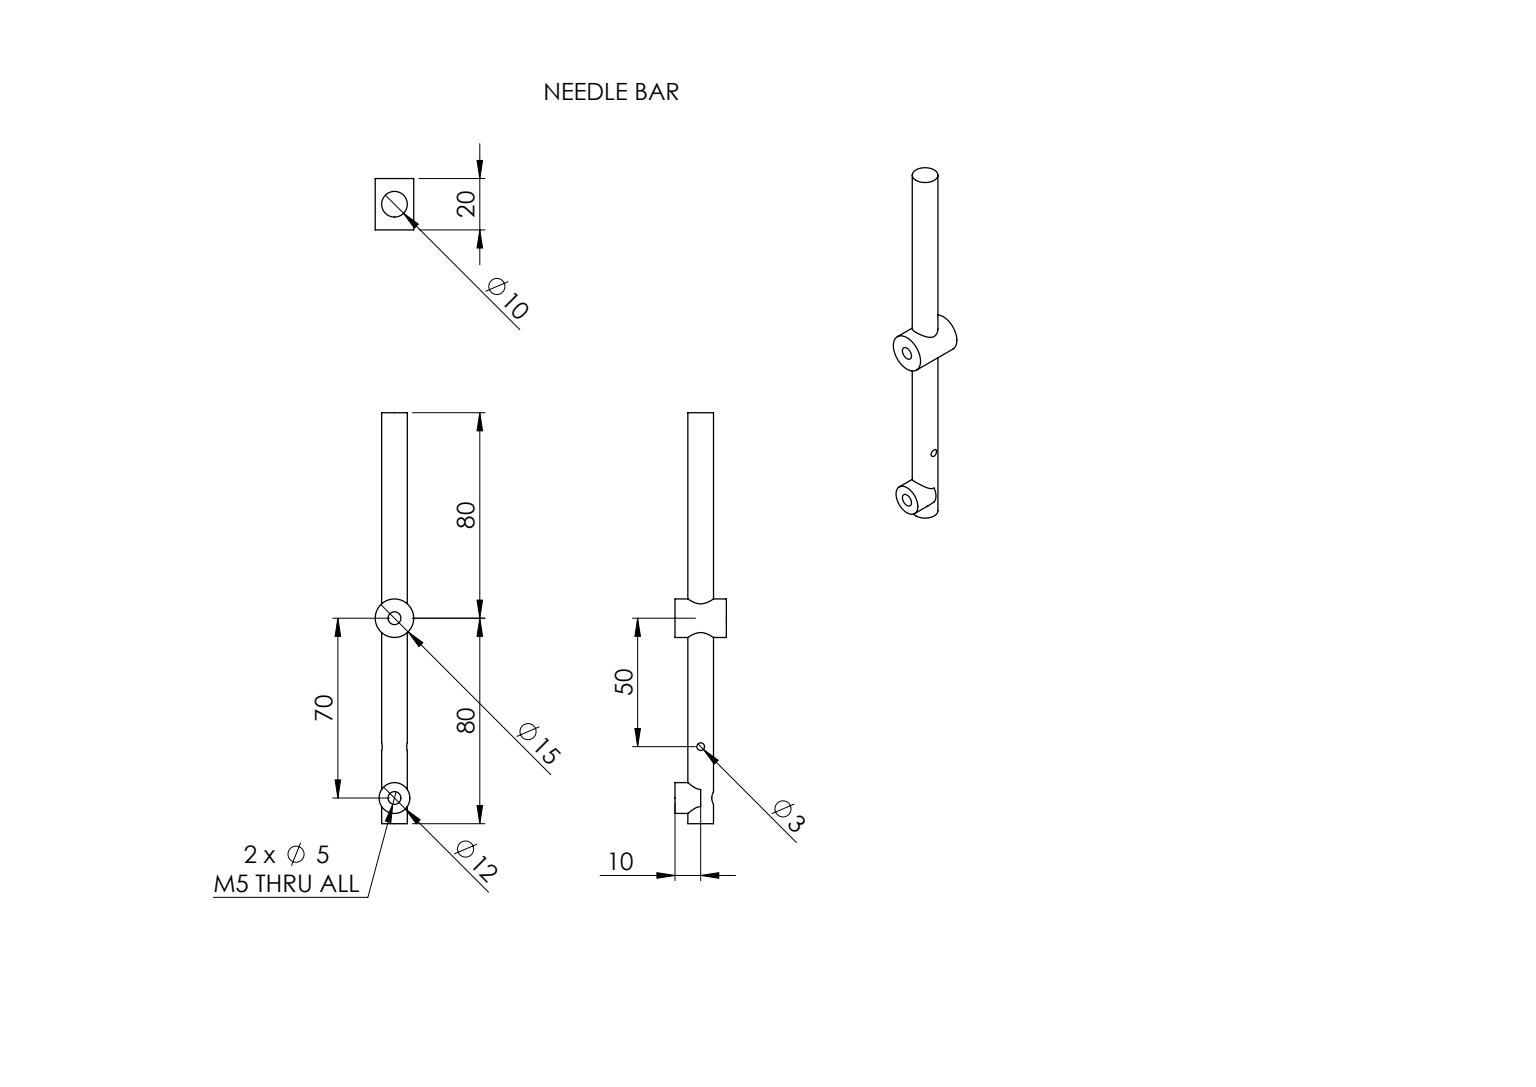
ISO-10303-21;
HEADER;
FILE_DESCRIPTION (('STEP AP214'),
    '1' );
FILE_NAME ('Needle Bar.step',
    '2026-10-25T11:00:22',
    ( '' ),
    ( '' ),
    'SwSTEP 2.0',
    'SolidWorks 2026',
    '' );
FILE_SCHEMA (( 'AUTOMOTIVE_DESIGN' ));
ENDSEC;

DATA;
#4=CARTESIAN_POINT ( 'NONE',  ( 4.999998311775604165, -51.49999437258534130, 0.09894250604207632804 ) ) ;
#5=SHAPE_DEFINITION_REPRESENTATION ( #2134, #457 ) ;
#6=CYLINDRICAL_SURFACE ( 'NONE', #1532, 4.999999999999999112 ) ;
#7=CARTESIAN_POINT ( 'NONE',  ( -0.1736799743064503798, -76.00000000000005684, 5.000000000000000000 ) ) ;
#8=UNCERTAINTY_MEASURE_WITH_UNIT (LENGTH_MEASURE( 1.000000000000000082E-05 ), #1107, 'distance_accuracy_value', 'NONE');
#17=CARTESIAN_POINT ( 'NONE',  ( 0.3311419820765648669, -72.48349571540411773, -4.991687326893459620 ) ) ;
#18=CARTESIAN_POINT ( 'NONE',  ( 2.499999999999999556, 3.061616997868382648E-16, 10.00000000000000000 ) ) ;
#21=CARTESIAN_POINT ( 'NONE',  ( 4.769696007084727185, -50.19647014491117432, 1.499999999999993339 ) ) ;
#22=ADVANCED_FACE ( 'NONE', ( #937 ), #2745, .F. ) ;
#24=CARTESIAN_POINT ( 'NONE',  ( -4.828212536628694984, -50.75366254478191053, 1.300578314244078992 ) ) ;
#26=CARTESIAN_POINT ( 'NONE',  ( 3.061616997868384127E-16, -72.50000000000001421, 2.500000000000000444 ) ) ;
#29=EDGE_LOOP ( 'NONE', ( #3142, #458 ) ) ;
#33=ORIENTED_EDGE ( 'NONE', *, *, #1677, .F. ) ;
#34=CARTESIAN_POINT ( 'NONE',  ( 4.871330634494102974, -50.99215130299450038, -1.129198576418441791 ) ) ;
#39=CARTESIAN_POINT ( 'NONE',  ( -3.982914377913044479, -74.49364316089672400, 3.038300766938668573 ) ) ;
#41=CARTESIAN_POINT ( 'NONE',  ( -7.500000000000000000, -50.00000000000000000, -1.500000000000006439 ) ) ;
#43=DIRECTION ( 'NONE',  ( 1.000000000000000000, -0.000000000000000000, -0.000000000000000000 ) ) ;
#46=DIRECTION ( 'NONE',  ( 0.000000000000000000, 1.000000000000000000, 0.000000000000000000 ) ) ;
#47=AXIS2_PLACEMENT_3D ( 'NONE', #892, #615, #1900 ) ;
#49=CARTESIAN_POINT ( 'NONE',  ( -6.610444160707455418E-15, -72.50000000000009948, -5.000000000000047962 ) ) ;
#51=CARTESIAN_POINT ( 'NONE',  ( 4.977204064302565456, -51.42262508310333402, -0.4855051584829146449 ) ) ;
#53=CIRCLE ( 'NONE', #2065, 4.999999999999999112 ) ;
#54=ADVANCED_FACE ( 'NONE', ( #463, #744 ), #700, .T. ) ;
#55=CARTESIAN_POINT ( 'NONE',  ( -0.3471650268615569246, -75.99247303379605967, 4.990975288187767589 ) ) ;
#57=CARTESIAN_POINT ( 'NONE',  ( 0.000000000000000000, 0.000000000000000000, 10.00000000000000000 ) ) ;
#59=EDGE_CURVE ( 'NONE', #1569, #129, #2568, .T. ) ;
#62=ORIENTED_EDGE ( 'NONE', *, *, #59, .F. ) ;
#63=CARTESIAN_POINT ( 'NONE',  ( 8.572527594031472993E-15, -70.00000000000000000, 10.00000000000000000 ) ) ;
#64=CARTESIAN_POINT ( 'NONE',  ( -2.499999999999995559, -70.00000000000000000, 0.000000000000000000 ) ) ;
#65=CARTESIAN_POINT ( 'NONE',  ( 4.964478897467096807, -5.622442520179988357, 0.6821754209311353678 ) ) ;
#68=CARTESIAN_POINT ( 'NONE',  ( -0.6778607859896496057, 7.476644527972223564, 4.965157125901431101 ) ) ;
#70=ORIENTED_EDGE ( 'NONE', *, *, #2414, .T. ) ;
#72=ADVANCED_FACE ( 'NONE', ( #1264 ), #1017, .F. ) ;
#79=CARTESIAN_POINT ( 'NONE',  ( 8.572527594031472993E-15, -70.00000000000000000, 10.00000000000000000 ) ) ;
#81=CARTESIAN_POINT ( 'NONE',  ( 4.966432541228214426, 5.620714496023337503, -0.6691698110145376521 ) ) ;
#82=CARTESIAN_POINT ( 'NONE',  ( 4.821318589555972700, -5.745344196342314191, 1.334996645354991074 ) ) ;
#84=VERTEX_POINT ( 'NONE', #2265 ) ;
#85=CYLINDRICAL_SURFACE ( 'NONE', #3102, 2.499999999999999556 ) ;
#86=AXIS2_PLACEMENT_3D ( 'NONE', #2225, #1782, #1240 ) ;
#89=CARTESIAN_POINT ( 'NONE',  ( -2.483686021788606091, -70.33016769071190311, -4.339668646282463627 ) ) ;
#90=CIRCLE ( 'NONE', #990, 6.000000000000001776 ) ;
#92=ORIENTED_EDGE ( 'NONE', *, *, #2004, .F. ) ;
#94=CARTESIAN_POINT ( 'NONE',  ( -0.8154661022227107647, -67.63113994865679501, -4.935425033279029705 ) ) ;
#96=FACE_OUTER_BOUND ( 'NONE', #2631, .T. ) ;
#97=VERTEX_POINT ( 'NONE', #26 ) ;
#98=EDGE_CURVE ( 'NONE', #842, #2258, #2815, .T. ) ;
#100=CARTESIAN_POINT ( 'NONE',  ( 2.543133226181223616, 7.061565991568797607, 4.317068135836759524 ) ) ;
#101=CARTESIAN_POINT ( 'NONE',  ( -0.3480864936855371794, -64.00754952754900273, 4.990948402655851268 ) ) ;
#103=CARTESIAN_POINT ( 'NONE',  ( -4.327080376399232264, 6.129587957101251483, -2.525419289280399049 ) ) ;
#105=ADVANCED_FACE ( 'NONE', ( #527 ), #307, .F. ) ;
#111=ORIENTED_EDGE ( 'NONE', *, *, #929, .T. ) ;
#112=DIRECTION ( 'NONE',  ( 1.000000000000000000, 0.000000000000000000, 0.000000000000000000 ) ) ;
#116=CARTESIAN_POINT ( 'NONE',  ( 8.572527594031472993E-15, -70.00000000000000000, 10.00000000000000000 ) ) ;
#118=CARTESIAN_POINT ( 'NONE',  ( 4.728889495302424528, 5.823500886956166411, 1.655898480698586139 ) ) ;
#123=VERTEX_POINT ( 'NONE', #544 ) ;
#128=CARTESIAN_POINT ( 'NONE',  ( 0.8153798621788117540, -67.63100920925315052, -4.935481307755256175 ) ) ;
#129=VERTEX_POINT ( 'NONE', #509 ) ;
#130=CARTESIAN_POINT ( 'NONE',  ( 0.000000000000000000, -80.00000000000000000, 4.999999999999999112 ) ) ;
#133=CARTESIAN_POINT ( 'NONE',  ( -4.964478897467096807, 5.622442520179988357, 0.6821754209311353678 ) ) ;
#135=EDGE_LOOP ( 'NONE', ( #2013, #111, #33, #444, #818, #2129 ) ) ;
#142=CARTESIAN_POINT ( 'NONE',  ( 0.000000000000000000, 0.000000000000000000, 10.00000000000000000 ) ) ;
#143=DIRECTION ( 'NONE',  ( 0.000000000000000000, -0.000000000000000000, 1.000000000000000000 ) ) ;
#144=ORIENTED_EDGE ( 'NONE', *, *, #2783, .T. ) ;
#145=CIRCLE ( 'NONE', #415, 4.999999999999999112 ) ;
#148=CARTESIAN_POINT ( 'NONE',  ( -3.971589419094359030, -6.365665093354385462, -3.054047635831909524 ) ) ;
#151=ORIENTED_EDGE ( 'NONE', *, *, #320, .T. ) ;
#154=VECTOR ( 'NONE', #1851, 1000.000000000000000 ) ;
#155=CARTESIAN_POINT ( 'NONE',  ( 0.000000000000000000, 0.000000000000000000, -10.00000000000000000 ) ) ;
#158=CARTESIAN_POINT ( 'NONE',  ( 7.500000000000000000, 9.184850993605147944E-16, 10.00000000000000000 ) ) ;
#160=CARTESIAN_POINT ( 'NONE',  ( 4.823113930341509814, -73.57101484999542151, 1.361197559098670462 ) ) ;
#162=CARTESIAN_POINT ( 'NONE',  ( -4.997074555615626856, -48.50966683676461599, -0.1965204501117691904 ) ) ;
#165=ADVANCED_FACE ( 'NONE', ( #1515, #3069 ), #289, .T. ) ;
#170=CARTESIAN_POINT ( 'NONE',  ( -4.999999999999999112, -73.31662479035540514, 0.000000000000000000 ) ) ;
#171=CARTESIAN_POINT ( 'NONE',  ( -5.999999999999992895, -70.00000000000000000, 0.000000000000000000 ) ) ;
#172=ORIENTED_EDGE ( 'NONE', *, *, #2667, .F. ) ;
#173=CARTESIAN_POINT ( 'NONE',  ( 0.1736799743064505464, -64.00000000000000000, 5.000000000000000000 ) ) ;
#177=CARTESIAN_POINT ( 'NONE',  ( 0.6967678811844650877, -75.96197462185259042, 4.954315763534759220 ) ) ;
#178=CARTESIAN_POINT ( 'NONE',  ( -4.769696007084725409, -50.00000000000000000, -1.500000000000006439 ) ) ;
#180=CARTESIAN_POINT ( 'NONE',  ( 4.784663389310397363, -49.60983055069853265, -1.451689076663209566 ) ) ;
#183=EDGE_LOOP ( 'NONE', ( #2116, #763, #2764, #874, #2899, #62, #1341 ) ) ;
#185=CARTESIAN_POINT ( 'NONE',  ( 1.259284006377631604, -72.16577835674955566, -4.840859579833913351 ) ) ;
#187=ORIENTED_EDGE ( 'NONE', *, *, #2783, .F. ) ;
#188=CARTESIAN_POINT ( 'NONE',  ( 1.181079518071022826E-19, -64.00000000000000000, 4.999999999999999112 ) ) ;
#192=CARTESIAN_POINT ( 'NONE',  ( -4.977204064302565456, -48.57737491689668730, -0.4855051584829146449 ) ) ;
#193=VECTOR ( 'NONE', #1958, 1000.000000000000000 ) ;
#195=CARTESIAN_POINT ( 'NONE',  ( 4.769696007084728073, -49.90173799037950886, 1.499999999999994449 ) ) ;
#197=FACE_OUTER_BOUND ( 'NONE', #689, .T. ) ;
#201=CARTESIAN_POINT ( 'NONE',  ( 6.000000000000010658, -70.00000000000000000, 0.000000000000000000 ) ) ;
#205=AXIS2_PLACEMENT_3D ( 'NONE', #2839, #2602, #2103 ) ;
#208=CARTESIAN_POINT ( 'NONE',  ( 4.999999999999999112, -73.31662479035541935, 0.000000000000000000 ) ) ;
#211=CARTESIAN_POINT ( 'NONE',  ( 4.793458659903279795, -49.51492518266869780, 1.422772306546142174 ) ) ;
#213=ADVANCED_FACE ( 'NONE', ( #2558, #772 ), #1795, .T. ) ;
#216=VERTEX_POINT ( 'NONE', #1535 ) ;
#218=CARTESIAN_POINT ( 'NONE',  ( 3.078327448814686562, -6.845130131842670274, -3.953084837412474517 ) ) ;
#219=( BOUNDED_CURVE ( )  B_SPLINE_CURVE ( 3, ( #377, #1897, #2151, #343 ),
 .UNSPECIFIED., .F., .F. ) 
 B_SPLINE_CURVE_WITH_KNOTS ( ( 4, 4 ),
 ( 3.141592653589794448, 4.712388980384689674 ),
 .UNSPECIFIED. ) 
 CURVE ( )  GEOMETRIC_REPRESENTATION_ITEM ( )  RATIONAL_B_SPLINE_CURVE ( ( 1.000000000000000000, 0.8047378541243652705, 0.8047378541243652705, 1.000000000000000000 ) ) 
 REPRESENTATION_ITEM ( '' )  );
#220=FACE_OUTER_BOUND ( 'NONE', #2600, .T. ) ;
#224=FACE_OUTER_BOUND ( 'NONE', #3125, .T. ) ;
#226=CARTESIAN_POINT ( 'NONE',  ( 4.769696007084729850, -50.00000000000000000, 1.499999999999994449 ) ) ;
#230=EDGE_CURVE ( 'NONE', #2611, #2101, #2545, .T. ) ;
#232=B_SPLINE_CURVE_WITH_KNOTS ( 'NONE', 3,
 ( #734, #2454, #2734, #180, #2224, #1192, #3011, #1751, #2761, #497, #2206, #3211, #468, #2748, #2964, #2268, #1506, #2517, #2503, #242, #1473, #3275, #2469, #211, #1938, #2720, #195, #226 ),
 .UNSPECIFIED., .F., .F.,
 ( 4, 2, 2, 2, 2, 2, 2, 2, 2, 2, 2, 2, 2, 4 ),
 ( 0.000000000000000000, 0.0002948077093299257545, 0.0005896154186598515090, 0.0008844231279897772635, 0.001179230837319703018, 0.001768846255979540866, 0.002358461674639378714, 0.002653269383969297963, 0.002948077093299216345, 0.003537692511959054844, 0.003832500221288973660, 0.004127307930618892041, 0.004422115639948811724, 0.004716923349278730540 ),
 .UNSPECIFIED. ) ;
#233=CARTESIAN_POINT ( 'NONE',  ( -4.476097271599867256, -65.99976937466333027, 2.250477508087396661 ) ) ;
#239=CIRCLE ( 'NONE', #570, 2.500000000000000000 ) ;
#240=CARTESIAN_POINT ( 'NONE',  ( 8.572527594031472993E-15, -70.00000000000000000, 0.000000000000000000 ) ) ;
#242=CARTESIAN_POINT ( 'NONE',  ( 4.871060595381011993, -49.00914020874981247, 1.130390421582378124 ) ) ;
#249=CARTESIAN_POINT ( 'NONE',  ( 4.793596727855903517, -50.48644371210733084, -1.422310562379361487 ) ) ;
#251=CARTESIAN_POINT ( 'NONE',  ( 4.666223265025314149, -5.872199985543652190, 1.803446265377422364 ) ) ;
#254=CARTESIAN_POINT ( 'NONE',  ( 3.061616997868384127E-16, -67.50000000000000000, 2.500000000000000444 ) ) ;
#260=ORIENTED_EDGE ( 'NONE', *, *, #511, .T. ) ;
#262=CARTESIAN_POINT ( 'NONE',  ( 1.116875426047833963, -72.24257843717799688, -4.876070537812395855 ) ) ;
#264=CARTESIAN_POINT ( 'NONE',  ( -7.500000000000000000, 0.000000000000000000, -10.00000000000000000 ) ) ;
#265=CARTESIAN_POINT ( 'NONE',  ( -0.6766787981060014001, -7.476722154948000743, 4.965272001127371659 ) ) ;
#268=CARTESIAN_POINT ( 'NONE',  ( 5.000001686767464371, -51.50000562255823411, -0.09877180560914068652 ) ) ;
#269=CARTESIAN_POINT ( 'NONE',  ( -4.325820249441205689, -65.83546891105626742, 2.526170042365371682 ) ) ;
#270=CARTESIAN_POINT ( 'NONE',  ( -4.793520869840776299, -50.48574331923479264, -1.422568331971221456 ) ) ;
#272=DIRECTION ( 'NONE',  ( 1.000000000000000000, -0.000000000000000000, -0.000000000000000000 ) ) ;
#281=CARTESIAN_POINT ( 'NONE',  ( 0.000000000000000000, -7.500000000000000000, 4.999999999999999112 ) ) ;
#284=CARTESIAN_POINT ( 'NONE',  ( 4.769696007084729850, -50.00000000000000000, 1.499999999999994449 ) ) ;
#286=ORIENTED_EDGE ( 'NONE', *, *, #755, .F. ) ;
#287=CARTESIAN_POINT ( 'NONE',  ( -4.871328134482659777, -50.99213922289512624, -1.129209473734892777 ) ) ;
#288=FACE_OUTER_BOUND ( 'NONE', #2430, .T. ) ;
#289=PLANE ( 'NONE',  #517 ) ;
#291=EDGE_CURVE ( 'NONE', #1132, #1384, #2523, .T. ) ;
#296=AXIS2_PLACEMENT_3D ( 'NONE', #3015, #539, #1547 ) ;
#297=EDGE_CURVE ( 'NONE', #2166, #335, #90, .T. ) ;
#299=CARTESIAN_POINT ( 'NONE',  ( -7.500000000000000000, -50.00000000000000000, 1.499999999999994449 ) ) ;
#301=CARTESIAN_POINT ( 'NONE',  ( 4.977300154039397739, -51.42297266766095021, 0.4847224211361968460 ) ) ;
#304=AXIS2_PLACEMENT_3D ( 'NONE', #1584, #565, #1317 ) ;
#305=CARTESIAN_POINT ( 'NONE',  ( -4.858119196087239189, -73.52168444273505088, 1.194558663167261781 ) ) ;
#307=PLANE ( 'NONE',  #836 ) ;
#316=CARTESIAN_POINT ( 'NONE',  ( 2.500000000000004441, -71.46446609406727646, -1.464466094067262025 ) ) ;
#318=AXIS2_PLACEMENT_3D ( 'NONE', #2727, #459, #1218 ) ;
#319=CARTESIAN_POINT ( 'NONE',  ( 4.985720285031673527, -51.45180769512853658, -0.3898302721915644087 ) ) ;
#320=EDGE_CURVE ( 'NONE', #1146, #2520, #1308, .T. ) ;
#324=CARTESIAN_POINT ( 'NONE',  ( -4.769696007084725409, -50.00000000000000000, -1.500000000000006439 ) ) ;
#325=DIRECTION ( 'NONE',  ( 1.000000000000000000, 0.000000000000000000, 0.000000000000000000 ) ) ;
#328=CARTESIAN_POINT ( 'NONE',  ( 2.500000000000008438, -70.00000000000000000, -4.330127018922187432 ) ) ;
#331=CARTESIAN_POINT ( 'NONE',  ( 0.000000000000000000, -80.00000000000000000, 0.000000000000000000 ) ) ;
#332=CARTESIAN_POINT ( 'NONE',  ( 4.476439251420855747, 6.019721759973592157, 2.250752599798611975 ) ) ;
#333=CARTESIAN_POINT ( 'NONE',  ( -1.375028959113679727, -64.14968884627424472, 4.819517586941451270 ) ) ;
#335=VERTEX_POINT ( 'NONE', #2320 ) ;
#336=CARTESIAN_POINT ( 'NONE',  ( -4.477156588595653020, 6.019182485879955635, 2.249288964509364774 ) ) ;
#343=CARTESIAN_POINT ( 'NONE',  ( -2.499999999999995559, -70.00000000000000000, 0.000000000000000000 ) ) ;
#344=CARTESIAN_POINT ( 'NONE',  ( -2.499999999999991118, -70.00000000000000000, 10.00000000000000000 ) ) ;
#346=ORIENTED_EDGE ( 'NONE', *, *, #411, .F. ) ;
#349=CARTESIAN_POINT ( 'NONE',  ( 3.321910197521175778, 6.728960966335735705, 3.750313380908745664 ) ) ;
#350=CARTESIAN_POINT ( 'NONE',  ( 4.769696007084729850, -50.00000000000000000, 1.499999999999994449 ) ) ;
#351=CARTESIAN_POINT ( 'NONE',  ( 6.121942914840092871E-16, -7.500000000000000000, -4.999999999999999112 ) ) ;
#354=AXIS2_PLACEMENT_3D ( 'NONE', #1287, #2089, #1073 ) ;
#356=VERTEX_POINT ( 'NONE', #49 ) ;
#358=CARTESIAN_POINT ( 'NONE',  ( -2.499999999999991118, -70.00000000000000000, -4.330127018922196314 ) ) ;
#359=CARTESIAN_POINT ( 'NONE',  ( 8.572527594031472993E-15, -70.00000000000000000, 10.00000000000000000 ) ) ;
#361=CARTESIAN_POINT ( 'NONE',  ( 6.122861072698252249E-16, -67.50000000000000000, -4.999999999999999112 ) ) ;
#363=CARTESIAN_POINT ( 'NONE',  ( 3.061616997868384127E-16, -72.50000000000001421, 2.500000000000000444 ) ) ;
#364=CARTESIAN_POINT ( 'NONE',  ( 1.985358491602502662, -68.47218767861880906, -4.589996648303077187 ) ) ;
#367=CARTESIAN_POINT ( 'NONE',  ( 3.971188403759415397, 6.365899760466498414, 3.054486213830300390 ) ) ;
#370=CARTESIAN_POINT ( 'NONE',  ( -3.966867482980610315, 6.368676471623262003, 3.060450018115215443 ) ) ;
#373=ORIENTED_EDGE ( 'NONE', *, *, #1718, .F. ) ;
#374=DIRECTION ( 'NONE',  ( 0.000000000000000000, 0.000000000000000000, 1.000000000000000000 ) ) ;
#375=( GEOMETRIC_REPRESENTATION_CONTEXT ( 3 ) GLOBAL_UNCERTAINTY_ASSIGNED_CONTEXT ( ( #8 ) ) GLOBAL_UNIT_ASSIGNED_CONTEXT ( ( #1107, #1543, #534 ) ) REPRESENTATION_CONTEXT ( 'NONE', 'WORKASPACE' ) );
#377=CARTESIAN_POINT ( 'NONE',  ( 3.061616997868384127E-16, -67.50000000000000000, 2.500000000000000444 ) ) ;
#378=LINE ( 'NONE', #1386, #2256 ) ;
#385=CARTESIAN_POINT ( 'NONE',  ( -3.077296587540346184, -6.845542784947758364, -3.953776968828220717 ) ) ;
#386=EDGE_CURVE ( 'NONE', #1748, #1911, #3165, .T. ) ;
#387=CARTESIAN_POINT ( 'NONE',  ( -4.999765607858179806, 5.590379590366716833, 0.3449705472529415728 ) ) ;
#389=EDGE_LOOP ( 'NONE', ( #1165, #392, #454 ) ) ;
#392=ORIENTED_EDGE ( 'NONE', *, *, #1084, .F. ) ;
#394=DIRECTION ( 'NONE',  ( -0.000000000000000000, -0.000000000000000000, 1.000000000000000000 ) ) ;
#395=LINE ( 'NONE', #1155, #422 ) ;
#397=CARTESIAN_POINT ( 'NONE',  ( -2.499999999999995559, -70.00000000000000000, 0.000000000000000000 ) ) ;
#400=CARTESIAN_POINT ( 'NONE',  ( -3.766216509439173965, 6.490735160851770047, 3.303865152441167297 ) ) ;
#401=EDGE_CURVE ( 'NONE', #2166, #2400, #1852, .T. ) ;
#404=AXIS2_PLACEMENT_3D ( 'NONE', #2772, #2300, #1519 ) ;
#406=CARTESIAN_POINT ( 'NONE',  ( 4.865239396163736352, -5.708012565174444219, -1.165122949380803741 ) ) ;
#411=EDGE_CURVE ( 'NONE', #1093, #651, #145, .T. ) ;
#412=DIRECTION ( 'NONE',  ( -0.000000000000000000, -0.000000000000000000, -1.000000000000000000 ) ) ;
#413=CARTESIAN_POINT ( 'NONE',  ( 1.541913646847672403, -68.00584954049281805, -4.762550599683263108 ) ) ;
#414=ORIENTED_EDGE ( 'NONE', *, *, #995, .T. ) ;
#415=AXIS2_PLACEMENT_3D ( 'NONE', #572, #1274, #519 ) ;
#416=CARTESIAN_POINT ( 'NONE',  ( -4.871117609892888112, -49.00886260987331866, 1.130144156083558560 ) ) ;
#418=CARTESIAN_POINT ( 'NONE',  ( -1.654328459400600471, -7.322002074975777930, -4.729864656991090932 ) ) ;
#421=ORIENTED_EDGE ( 'NONE', *, *, #2954, .T. ) ;
#422=VECTOR ( 'NONE', #2170, 1000.000000000000000 ) ;
#425=( GEOMETRIC_REPRESENTATION_CONTEXT ( 3 ) GLOBAL_UNCERTAINTY_ASSIGNED_CONTEXT ( ( #2296 ) ) GLOBAL_UNIT_ASSIGNED_CONTEXT ( ( #2905, #1350, #613 ) ) REPRESENTATION_CONTEXT ( 'NONE', 'WORKASPACE' ) );
#426=CARTESIAN_POINT ( 'NONE',  ( 3.326284669807233918, -6.726800191391157924, -3.746459129603366467 ) ) ;
#428=CARTESIAN_POINT ( 'NONE',  ( 3.982914377913047144, -65.50635683910327600, 3.038300766938665465 ) ) ;
#432=CARTESIAN_POINT ( 'NONE',  ( 1.698458751326837435, -75.76378408612910675, 4.714595771049563844 ) ) ;
#434=CARTESIAN_POINT ( 'NONE',  ( -4.828119302692784665, -49.24690690879460675, -1.300931117799746906 ) ) ;
#441=CARTESIAN_POINT ( 'NONE',  ( 1.654531499027267483, -71.88102071354902023, -4.719874665594111285 ) ) ;
#444=ORIENTED_EDGE ( 'NONE', *, *, #386, .F. ) ;
#448=CARTESIAN_POINT ( 'NONE',  ( 0.1739454948912135535, -76.00000000000001421, 4.999999999999999112 ) ) ;
#449=CARTESIAN_POINT ( 'NONE',  ( -4.769696007084725409, -49.90029503198832828, -1.500000000000006217 ) ) ;
#454=ORIENTED_EDGE ( 'NONE', *, *, #1643, .F. ) ;
#456=CARTESIAN_POINT ( 'NONE',  ( 1.653246020961511187, -7.322320024462306343, -4.730368990601279577 ) ) ;
#457=SHAPE_REPRESENTATION ( 'Needle Bar', ( #1692 ), #1164 ) ;
#458=ORIENTED_EDGE ( 'NONE', *, *, #1898, .F. ) ;
#459=DIRECTION ( 'NONE',  ( 0.000000000000000000, 0.000000000000000000, 1.000000000000000000 ) ) ;
#463=FACE_BOUND ( 'NONE', #2805, .T. ) ;
#465=CARTESIAN_POINT ( 'NONE',  ( -4.985625624127048461, -48.54851733604390773, 0.3909128500499727821 ) ) ;
#466=VECTOR ( 'NONE', #2091, 1000.000000000000000 ) ;
#468=CARTESIAN_POINT ( 'NONE',  ( 4.999974214802088035, -48.50008595066712047, -0.1976414581757740541 ) ) ;
#471=ORIENTED_EDGE ( 'NONE', *, *, #568, .F. ) ;
#473=EDGE_CURVE ( 'NONE', #1139, #1195, #1896, .T. ) ;
#479=DIRECTION ( 'NONE',  ( 0.000000000000000000, 0.000000000000000000, 1.000000000000000000 ) ) ;
#480=STYLED_ITEM('',(#3321),#2670);
#482=EDGE_CURVE ( 'NONE', #1748, #2258, #2467, .T. ) ;
#486=CARTESIAN_POINT ( 'NONE',  ( 8.572527594031472993E-15, -70.00000000000000000, 0.000000000000000000 ) ) ;
#490=CARTESIAN_POINT ( 'NONE',  ( -3.984264206898689320, -65.50759766373489867, 3.036427941355733129 ) ) ;
#492=LINE ( 'NONE', #1970, #1319 ) ;
#494=CARTESIAN_POINT ( 'NONE',  ( 4.999999999999999112, -73.31662479035543356, 0.3546751931833549421 ) ) ;
#495=CARTESIAN_POINT ( 'NONE',  ( 2.500000000000000000, 3.061616997868383141E-16, -10.00000000000000000 ) ) ;
#497=CARTESIAN_POINT ( 'NONE',  ( 4.916101592540525367, -48.80164085375129446, -0.9229043554563169938 ) ) ;
#503=FACE_OUTER_BOUND ( 'NONE', #2122, .T. ) ;
#505=CARTESIAN_POINT ( 'NONE',  ( 0.000000000000000000, -60.00000000000000000, 0.000000000000000000 ) ) ;
#506=PRODUCT_DEFINITION_CONTEXT ( 'detailed design', #1636, 'design' ) ;
#509=CARTESIAN_POINT ( 'NONE',  ( -1.181079518071022826E-19, -76.00000000000001421, 4.999999999999999112 ) ) ;
#510=CIRCLE ( 'NONE', #354, 6.000000000000001776 ) ;
#511=EDGE_CURVE ( 'NONE', #810, #1748, #1991, .T. ) ;
#512=DIRECTION ( 'NONE',  ( 0.000000000000000000, -0.000000000000000000, 1.000000000000000000 ) ) ;
#515=FACE_BOUND ( 'NONE', #2326, .T. ) ;
#516=DIRECTION ( 'NONE',  ( 0.000000000000000000, -1.000000000000000000, 0.000000000000000000 ) ) ;
#517=AXIS2_PLACEMENT_3D ( 'NONE', #2283, #2527, #2034 ) ;
#519=DIRECTION ( 'NONE',  ( 0.000000000000000000, 0.000000000000000000, 1.000000000000000000 ) ) ;
#524=CARTESIAN_POINT ( 'NONE',  ( 4.999765607858179806, -5.590379590366716833, 0.3449705472529415728 ) ) ;
#525=CARTESIAN_POINT ( 'NONE',  ( -4.793458659903279795, -50.48507481733130220, 1.422772306546142174 ) ) ;
#527=FACE_OUTER_BOUND ( 'NONE', #1943, .T. ) ;
#532=ORIENTED_EDGE ( 'NONE', *, *, #297, .T. ) ;
#534=( NAMED_UNIT ( * ) SI_UNIT ( $, .STERADIAN. ) SOLID_ANGLE_UNIT ( ) );
#535=CARTESIAN_POINT ( 'NONE',  ( 0.000000000000000000, 0.000000000000000000, -10.00000000000000000 ) ) ;
#537=CARTESIAN_POINT ( 'NONE',  ( 0.000000000000000000, -7.500000000000000000, 4.999999999999999112 ) ) ;
#539=DIRECTION ( 'NONE',  ( -0.000000000000000000, -0.000000000000000000, -1.000000000000000000 ) ) ;
#541=CARTESIAN_POINT ( 'NONE',  ( 0.000000000000000000, -80.00000000000000000, 4.999999999999999112 ) ) ;
#544=CARTESIAN_POINT ( 'NONE',  ( 2.500000000000008882, -70.00000000000000000, 10.00000000000000000 ) ) ;
#550=ORIENTED_EDGE ( 'NONE', *, *, #1924, .F. ) ;
#553=EDGE_CURVE ( 'NONE', #2101, #2520, #232, .T. ) ;
#557=CARTESIAN_POINT ( 'NONE',  ( 6.121942914840092871E-16, -7.500000000000000000, -4.999999999999999112 ) ) ;
#565=DIRECTION ( 'NONE',  ( -0.000000000000000000, -0.000000000000000000, -1.000000000000000000 ) ) ;
#568=EDGE_CURVE ( 'NONE', #2400, #3266, #1678, .T. ) ;
#570=AXIS2_PLACEMENT_3D ( 'NONE', #1402, #1971, #953 ) ;
#572=CARTESIAN_POINT ( 'NONE',  ( 0.000000000000000000, -80.00000000000000000, 0.000000000000000000 ) ) ;
#573=ORIENTED_EDGE ( 'NONE', *, *, #1778, .F. ) ;
#574=CARTESIAN_POINT ( 'NONE',  ( 4.916186798144710934, -51.19881560760884298, 0.9225820817148873143 ) ) ;
#577=CARTESIAN_POINT ( 'NONE',  ( -4.945777185212984151, -51.30992422645292805, -0.7564652374250301348 ) ) ;
#579=ORIENTED_EDGE ( 'NONE', *, *, #2417, .F. ) ;
#584=DIRECTION ( 'NONE',  ( -0.000000000000000000, -0.000000000000000000, -1.000000000000000000 ) ) ;
#586=CARTESIAN_POINT ( 'NONE',  ( 4.956114419722681852, 5.629162412197389109, 0.6822959203856070465 ) ) ;
#587=CARTESIAN_POINT ( 'NONE',  ( -2.594030646330689915, -64.58156784093502267, 4.286313293421136983 ) ) ;
#590=STYLED_ITEM ( 'NONE', ( #1305 ), #3218 ) ;
#591=CARTESIAN_POINT ( 'NONE',  ( -3.071765256614000794, 6.848070662608381376, 3.958153484541630629 ) ) ;
#597=EDGE_LOOP ( 'NONE', ( #2359, #1846, #1716, #2737 ) ) ;
#598=CARTESIAN_POINT ( 'NONE',  ( -2.369138637566329475, -69.18494310611589526, -4.403673215483854264 ) ) ;
#602=CARTESIAN_POINT ( 'NONE',  ( -2.499999999999995559, -70.00000000000000000, 0.000000000000000000 ) ) ;
#603=CARTESIAN_POINT ( 'NONE',  ( 3.769434200324356166, 6.488926209160664094, -3.300387065219955840 ) ) ;
#604=CARTESIAN_POINT ( 'NONE',  ( -4.769696007084725409, -50.00000000000000000, -1.500000000000006439 ) ) ;
#607=CARTESIAN_POINT ( 'NONE',  ( -2.262527220957939456, 7.157552900320828471, -4.471083064257649120 ) ) ;
#609=ADVANCED_FACE ( 'NONE', ( #224 ), #792, .T. ) ;
#612=ORIENTED_EDGE ( 'NONE', *, *, #2025, .F. ) ;
#613=( NAMED_UNIT ( * ) SI_UNIT ( $, .STERADIAN. ) SOLID_ANGLE_UNIT ( ) );
#615=DIRECTION ( 'NONE',  ( 0.000000000000000000, 0.000000000000000000, 1.000000000000000000 ) ) ;
#621=CARTESIAN_POINT ( 'NONE',  ( 3.078112602769041306, 6.845324219060942461, 3.953457562721318652 ) ) ;
#623=CARTESIAN_POINT ( 'NONE',  ( 2.500000000000004441, -70.00000000000000000, 0.000000000000000000 ) ) ;
#625=CARTESIAN_POINT ( 'NONE',  ( -1.653246020961511187, 7.322320024462306343, -4.730368990601279577 ) ) ;
#628=ORIENTED_EDGE ( 'NONE', *, *, #1396, .F. ) ;
#632=CARTESIAN_POINT ( 'NONE',  ( 0.000000000000000000, -80.00000000000000000, 0.000000000000000000 ) ) ;
#633=DIRECTION ( 'NONE',  ( 1.000000000000000000, 0.000000000000000000, 0.000000000000000000 ) ) ;
#635=CARTESIAN_POINT ( 'NONE',  ( 2.500000000000008438, -70.00000000000000000, -4.330127018922187432 ) ) ;
#637=ORIENTED_EDGE ( 'NONE', *, *, #1230, .F. ) ;
#640=CARTESIAN_POINT ( 'NONE',  ( -0.6733179620838674051, -7.471617105689219329, -4.957340513892267708 ) ) ;
#641=CARTESIAN_POINT ( 'NONE',  ( -4.481108542057384625, 6.016226048536217341, -2.241414944841849888 ) ) ;
#644=CIRCLE ( 'NONE', #3010, 6.000000000000001776 ) ;
#645=ORIENTED_EDGE ( 'NONE', *, *, #2417, .T. ) ;
#646=CARTESIAN_POINT ( 'NONE',  ( -2.369101981968370740, -70.81463507927145429, -4.403671262993352542 ) ) ;
#647=EDGE_LOOP ( 'NONE', ( #532, #1819 ) ) ;
#648=CARTESIAN_POINT ( 'NONE',  ( -1.115681787891026344, -67.75684662697969429, -4.876336675329124404 ) ) ;
#650=CARTESIAN_POINT ( 'NONE',  ( 0.000000000000000000, -80.00000000000000000, 0.000000000000000000 ) ) ;
#651=VERTEX_POINT ( 'NONE', #2067 ) ;
#655=CARTESIAN_POINT ( 'NONE',  ( -5.000292928619530564, -5.589907940605836956, -0.3348667354298545673 ) ) ;
#656=DIRECTION ( 'NONE',  ( 1.000000000000000000, 0.000000000000000000, 0.000000000000000000 ) ) ;
#658=EDGE_LOOP ( 'NONE', ( #286, #1842 ) ) ;
#665=ORIENTED_EDGE ( 'NONE', *, *, #1677, .T. ) ;
#666=CARTESIAN_POINT ( 'NONE',  ( -5.000001686767464371, -48.49999437744178010, -0.09877180560914068652 ) ) ;
#668=CARTESIAN_POINT ( 'NONE',  ( -1.338285735402328314, -7.387167716089622083, -4.829375120343072147 ) ) ;
#669=B_SPLINE_CURVE_WITH_KNOTS ( 'NONE', 3,
 ( #1420, #2188, #1387, #2403, #128, #864, #413, #3161, #364, #877, #1172, #2387, #2890, #2922, #1863, #635 ),
 .UNSPECIFIED., .F., .F.,
 ( 4, 2, 2, 2, 2, 2, 2, 4 ),
 ( 0.01192236024948129317, 0.01241818132785782632, 0.01291400240623435947, 0.01390564456298742750, 0.01440146564136396065, 0.01489728671974049554, 0.01539310779811702869, 0.01588892887649356184 ),
 .UNSPECIFIED. ) ;
#672=EDGE_CURVE ( 'NONE', #1979, #1630, #2893, .T. ) ;
#678=EDGE_LOOP ( 'NONE', ( #784, #1680 ) ) ;
#679=CARTESIAN_POINT ( 'NONE',  ( 4.815265823182746097, -66.41952955260356362, 1.356348383020189230 ) ) ;
#683=AXIS2_PLACEMENT_3D ( 'NONE', #1844, #891, #876 ) ;
#684=CARTESIAN_POINT ( 'NONE',  ( -4.871330634494102974, -49.00784869700550672, -1.129198576418441791 ) ) ;
#689=EDGE_LOOP ( 'NONE', ( #1211, #2505, #1101, #92, #1893, #1269, #815, #144, #2074, #1732, #2092 ) ) ;
#690=CIRCLE ( 'NONE', #791, 2.500000000000000444 ) ;
#693=DIRECTION ( 'NONE',  ( 0.000000000000000000, 0.000000000000000000, -1.000000000000000000 ) ) ;
#700=PLANE ( 'NONE',  #2102 ) ;
#701=CARTESIAN_POINT ( 'NONE',  ( -4.782644271597511043, -49.60515857921176064, 1.460283231774381907 ) ) ;
#710=ADVANCED_FACE ( 'NONE', ( #1300 ), #2316, .F. ) ;
#714=CARTESIAN_POINT ( 'NONE',  ( -5.999999999999992895, -70.00000000000000000, 10.00000000000000000 ) ) ;
#721=VERTEX_POINT ( 'NONE', #495 ) ;
#729=VECTOR ( 'NONE', #820, 1000.000000000000000 ) ;
#734=CARTESIAN_POINT ( 'NONE',  ( 4.769696007084725409, -50.00000000000000000, -1.500000000000006439 ) ) ;
#740=AXIS2_PLACEMENT_3D ( 'NONE', #116, #1623, #2876 ) ;
#741=DIRECTION ( 'NONE',  ( 0.000000000000000000, 0.000000000000000000, -1.000000000000000000 ) ) ;
#744=FACE_OUTER_BOUND ( 'NONE', #647, .T. ) ;
#746=B_SPLINE_CURVE_WITH_KNOTS ( 'NONE', 3,
 ( #1376, #2392, #1868, #2638, #2353, #2877, #100, #621, #349, #3113, #367, #3132, #332, #118, #2604, #1109, #586, #867, #1338, #1590, #81, #1090, #2126, #2106, #1850, #2862, #603, #1607, #1357, #3064, #2765, #800, #2275, #1770, #2777, #1577, #1527, #816, #1062, #2075 ),
 .UNSPECIFIED., .F., .F.,
 ( 4, 2, 2, 2, 2, 2, 2, 2, 2, 2, 2, 2, 2, 2, 2, 2, 2, 2, 2, 4 ),
 ( 0.000000000000000000, 0.001009991476537153501, 0.002019982953074307436, 0.003029974429611462239, 0.004039965906148617475, 0.005049957382685771844, 0.006059948859222927947, 0.007069940335760082316, 0.007574936074028659934, 0.008079931812297236685, 0.009089923288834390186, 0.01009991476537154195, 0.01110990624190869892, 0.01211989771844585242, 0.01312988919498300593, 0.01363488493325158528, 0.01413988067152016116, 0.01514987214805731987, 0.01565486788632589749, 0.01615986362459447684 ),
 .UNSPECIFIED. ) ;
#754=CARTESIAN_POINT ( 'NONE',  ( 4.945480083184111919, -51.30885859099010560, 0.7590239407556941265 ) ) ;
#755=EDGE_CURVE ( 'NONE', #3070, #721, #2000, .T. ) ;
#756=CARTESIAN_POINT ( 'NONE',  ( 1.334319281011194347, -7.387780498848168342, 4.830307711356911504 ) ) ;
#757=ADVANCED_FACE ( 'NONE', ( #1102 ), #3160, .F. ) ;
#758=DIRECTION ( 'NONE',  ( 0.000000000000000000, 1.000000000000000000, 0.000000000000000000 ) ) ;
#763=ORIENTED_EDGE ( 'NONE', *, *, #297, .F. ) ;
#764=LINE ( 'NONE', #2789, #2937 ) ;
#769=CARTESIAN_POINT ( 'NONE',  ( -1.373679055183323117, -75.85067040024597418, 4.819953665648757379 ) ) ;
#772=FACE_BOUND ( 'NONE', #678, .T. ) ;
#773=( BOUNDED_CURVE ( )  B_SPLINE_CURVE ( 3, ( #397, #2665, #1405, #2421 ),
 .UNSPECIFIED., .F., .T. ) 
 B_SPLINE_CURVE_WITH_KNOTS ( ( 4, 4 ),
 ( 4.712388980384689674, 6.283185307179586232 ),
 .UNSPECIFIED. ) 
 CURVE ( )  GEOMETRIC_REPRESENTATION_ITEM ( )  RATIONAL_B_SPLINE_CURVE ( ( 1.000000000000000000, 0.8047378541243649375, 0.8047378541243649375, 1.000000000000000000 ) ) 
 REPRESENTATION_ITEM ( '' )  );
#775=VECTOR ( 'NONE', #2055, 1000.000000000000000 ) ;
#782=DIRECTION ( 'NONE',  ( -0.000000000000000000, -0.000000000000000000, -1.000000000000000000 ) ) ;
#784=ORIENTED_EDGE ( 'NONE', *, *, #473, .F. ) ;
#785=CARTESIAN_POINT ( 'NONE',  ( 4.828119302692784665, -50.75309309120538614, -1.300931117799746906 ) ) ;
#788=DIRECTION ( 'NONE',  ( -0.000000000000000000, -0.000000000000000000, -1.000000000000000000 ) ) ;
#791=AXIS2_PLACEMENT_3D ( 'NONE', #2580, #879, #2621 ) ;
#792=PLANE ( 'NONE',  #1520 ) ;
#794=AXIS2_PLACEMENT_3D ( 'NONE', #3254, #1999, #741 ) ;
#795=ORIENTED_EDGE ( 'NONE', *, *, #2848, .T. ) ;
#800=CARTESIAN_POINT ( 'NONE',  ( 2.257837506661119154, 7.153666188643283519, -4.464160652961850495 ) ) ;
#802=ORIENTED_EDGE ( 'NONE', *, *, #1115, .T. ) ;
#803=CARTESIAN_POINT ( 'NONE',  ( -4.661216347248876346, -73.77919958324079630, 1.816027882404183114 ) ) ;
#805=CARTESIAN_POINT ( 'NONE',  ( -1.181079518071022826E-19, -76.00000000000001421, 4.999999999999999112 ) ) ;
#810=VERTEX_POINT ( 'NONE', #328 ) ;
#811=EDGE_CURVE ( 'NONE', #335, #2166, #1467, .T. ) ;
#814=CARTESIAN_POINT ( 'NONE',  ( -5.999999999999992895, -70.00000000000000000, 10.00000000000000000 ) ) ;
#815=ORIENTED_EDGE ( 'NONE', *, *, #2912, .F. ) ;
#816=CARTESIAN_POINT ( 'NONE',  ( 0.3369232893658926642, 7.494324649304657804, -4.991499248304590353 ) ) ;
#818=ORIENTED_EDGE ( 'NONE', *, *, #511, .F. ) ;
#819=DIRECTION ( 'NONE',  ( 0.000000000000000000, -1.000000000000000000, 0.000000000000000000 ) ) ;
#820=DIRECTION ( 'NONE',  ( -0.000000000000000000, -1.000000000000000000, -0.000000000000000000 ) ) ;
#821=VERTEX_POINT ( 'NONE', #863 ) ;
#829=CIRCLE ( 'NONE', #2682, 6.000000000000001776 ) ;
#831=CARTESIAN_POINT ( 'NONE',  ( 2.259265036967212481, -7.158401641891561695, 4.472413388026437175 ) ) ;
#833=ORIENTED_EDGE ( 'NONE', *, *, #3154, .T. ) ;
#836=AXIS2_PLACEMENT_3D ( 'NONE', #2313, #3274, #2573 ) ;
#840=CARTESIAN_POINT ( 'NONE',  ( -0.3347605109170348481, -72.48298187229545420, -4.991431073436380039 ) ) ;
#841=DIRECTION ( 'NONE',  ( -1.000000000000000000, 0.000000000000000000, 0.000000000000000000 ) ) ;
#842=VERTEX_POINT ( 'NONE', #2836 ) ;
#848=FILL_AREA_STYLE_COLOUR ( '', #2121 ) ;
#849=VECTOR ( 'NONE', #2481, 1000.000000000000000 ) ;
#850=CARTESIAN_POINT ( 'NONE',  ( -4.769696007084729850, -50.00000000000000000, 1.499999999999994449 ) ) ;
#851=CARTESIAN_POINT ( 'NONE',  ( 4.477156588595653020, -6.019182485879955635, 2.249288964509364774 ) ) ;
#852=DIRECTION ( 'NONE',  ( 1.000000000000000000, -0.000000000000000000, -0.000000000000000000 ) ) ;
#861=CARTESIAN_POINT ( 'NONE',  ( -0.3318670470563950814, -67.51651316714541906, -4.991680947004272006 ) ) ;
#863=CARTESIAN_POINT ( 'NONE',  ( -2.499999999999991562, -70.00000000000000000, 10.00000000000000000 ) ) ;
#864=CARTESIAN_POINT ( 'NONE',  ( 1.269654200241442377, -67.82150855935358891, -4.845952790443002201 ) ) ;
#866=CYLINDRICAL_SURFACE ( 'NONE', #3223, 6.000000000000001776 ) ;
#867=CARTESIAN_POINT ( 'NONE',  ( 4.990888858476322021, 5.598354044414833197, 0.3458703032855571791 ) ) ;
#871=CARTESIAN_POINT ( 'NONE',  ( -4.823237137747319103, 5.743727463073391881, -1.327965985491348588 ) ) ;
#874=ORIENTED_EDGE ( 'NONE', *, *, #568, .T. ) ;
#876=DIRECTION ( 'NONE',  ( 0.000000000000000000, 0.000000000000000000, -1.000000000000000000 ) ) ;
#877=CARTESIAN_POINT ( 'NONE',  ( 2.164733944603292493, -68.73913292587020862, -4.508175298354527349 ) ) ;
#879=DIRECTION ( 'NONE',  ( 0.000000000000000000, -1.000000000000000000, 0.000000000000000000 ) ) ;
#891=DIRECTION ( 'NONE',  ( -0.000000000000000000, -1.000000000000000000, -0.000000000000000000 ) ) ;
#892=CARTESIAN_POINT ( 'NONE',  ( 0.000000000000000000, 0.000000000000000000, -10.00000000000000000 ) ) ;
#896=CARTESIAN_POINT ( 'NONE',  ( -4.831975997384719612, -5.736714355192817472, -1.328626502536248699 ) ) ;
#902=CARTESIAN_POINT ( 'NONE',  ( -2.181554758577748387, -71.26329604159570863, -4.501186289107192096 ) ) ;
#903=VERTEX_POINT ( 'NONE', #2649 ) ;
#904=CARTESIAN_POINT ( 'NONE',  ( -1.260899024725782080, -67.83519155447288540, -4.840427811610033437 ) ) ;
#905=DIRECTION ( 'NONE',  ( 1.000000000000000000, 0.000000000000000000, 0.000000000000000000 ) ) ;
#908=DIRECTION ( 'NONE',  ( 1.000000000000000000, 0.000000000000000000, -0.000000000000000000 ) ) ;
#916=DIRECTION ( 'NONE',  ( 1.000000000000000000, 0.000000000000000000, 0.000000000000000000 ) ) ;
#917=ORIENTED_EDGE ( 'NONE', *, *, #2667, .T. ) ;
#920=DIRECTION ( 'NONE',  ( -0.000000000000000000, -0.000000000000000000, -1.000000000000000000 ) ) ;
#921=CARTESIAN_POINT ( 'NONE',  ( 3.117018002318638459, -75.13542606116712363, 3.922457828541068281 ) ) ;
#924=CARTESIAN_POINT ( 'NONE',  ( -4.930411998009738284, -5.651814738127338700, 0.8477781614216437500 ) ) ;
#925=EDGE_CURVE ( 'NONE', #651, #356, #2618, .T. ) ;
#929=EDGE_CURVE ( 'NONE', #2083, #2713, #1634, .T. ) ;
#931=CARTESIAN_POINT ( 'NONE',  ( 6.123233995736765296E-16, -80.00000000000000000, -4.999999999999999112 ) ) ;
#932=DIRECTION ( 'NONE',  ( 0.000000000000000000, 0.000000000000000000, 1.000000000000000000 ) ) ;
#935=CARTESIAN_POINT ( 'NONE',  ( 6.000000000000010658, -70.00000000000000000, 10.00000000000000000 ) ) ;
#936=DIRECTION ( 'NONE',  ( -0.000000000000000000, -1.000000000000000000, -0.000000000000000000 ) ) ;
#937=FACE_OUTER_BOUND ( 'NONE', #2646, .T. ) ;
#938=CARTESIAN_POINT ( 'NONE',  ( -4.828226831489238258, -49.24623717837067716, 1.300528505912509125 ) ) ;
#942=EDGE_CURVE ( 'NONE', #3014, #1569, #378, .T. ) ;
#947=AXIS2_PLACEMENT_3D ( 'NONE', #632, #1861, #1368 ) ;
#953=DIRECTION ( 'NONE',  ( -1.000000000000000000, 0.000000000000000000, 0.000000000000000000 ) ) ;
#957=CARTESIAN_POINT ( 'NONE',  ( -4.784702204231576772, -49.60930290693747935, -1.451562066005745999 ) ) ;
#964=CARTESIAN_POINT ( 'NONE',  ( 0.8162268732147681671, -72.36861614780602281, -4.935306302396404554 ) ) ;
#965=DIRECTION ( 'NONE',  ( -1.000000000000000000, 0.000000000000000000, 0.000000000000000000 ) ) ;
#967=CARTESIAN_POINT ( 'NONE',  ( 6.122861072698252249E-16, -67.50000000000000000, -4.999999999999999112 ) ) ;
#968=EDGE_CURVE ( 'NONE', #97, #1748, #2385, .T. ) ;
#971=CARTESIAN_POINT ( 'NONE',  ( 4.476097271599868144, -74.00023062533671236, 2.250477508087392220 ) ) ;
#979=CARTESIAN_POINT ( 'NONE',  ( 4.823237137747319103, -5.743727463073391881, -1.327965985491348588 ) ) ;
#980=VECTOR ( 'NONE', #3128, 1000.000000000000000 ) ;
#981=LINE ( 'NONE', #2447, #849 ) ;
#983=EDGE_CURVE ( 'NONE', #1926, #1036, #1773, .T. ) ;
#986=EDGE_CURVE ( 'NONE', #335, #3146, #1698, .T. ) ;
#990=AXIS2_PLACEMENT_3D ( 'NONE', #359, #2115, #325 ) ;
#995=EDGE_CURVE ( 'NONE', #821, #123, #1461, .T. ) ;
#998=CARTESIAN_POINT ( 'NONE',  ( -1.698458751326834992, -64.23621591387086482, 4.714595771049563844 ) ) ;
#999=CIRCLE ( 'NONE', #2057, 2.500000000000000000 ) ;
#1000=LINE ( 'NONE', #541, #1002 ) ;
#1002=VECTOR ( 'NONE', #758, 1000.000000000000000 ) ;
#1012=ORIENTED_EDGE ( 'NONE', *, *, #2852, .T. ) ;
#1013=CARTESIAN_POINT ( 'NONE',  ( 4.916102558146631551, -51.19836246274143576, -0.9228986618089604077 ) ) ;
#1014=CARTESIAN_POINT ( 'NONE',  ( -4.999999999999999112, -66.68337520964460907, 0.000000000000000000 ) ) ;
#1015=CARTESIAN_POINT ( 'NONE',  ( -2.592701047953011706, -75.41913213518454029, 4.287209529367745908 ) ) ;
#1017=CYLINDRICAL_SURFACE ( 'NONE', #2572, 2.500000000000000444 ) ;
#1020=ORIENTED_EDGE ( 'NONE', *, *, #98, .T. ) ;
#1021=CARTESIAN_POINT ( 'NONE',  ( 0.000000000000000000, -80.00000000000000000, -2.500000000000000444 ) ) ;
#1024=FACE_OUTER_BOUND ( 'NONE', #3097, .T. ) ;
#1028=CARTESIAN_POINT ( 'NONE',  ( 4.772823865982902092, -50.19777939995103111, -1.490154340647099174 ) ) ;
#1029=EDGE_CURVE ( 'NONE', #721, #3070, #239, .T. ) ;
#1036=VERTEX_POINT ( 'NONE', #158 ) ;
#1037=AXIS2_PLACEMENT_3D ( 'NONE', #2701, #2003, #2434 ) ;
#1040=CARTESIAN_POINT ( 'NONE',  ( -3.767802750538409295, -6.489812437959999514, 3.302060000734929446 ) ) ;
#1041=ORIENTED_EDGE ( 'NONE', *, *, #968, .T. ) ;
#1042=CARTESIAN_POINT ( 'NONE',  ( 4.871117609892888112, -50.99113739012668844, 1.130144156083558560 ) ) ;
#1043=EDGE_CURVE ( 'NONE', #3266, #2549, #1186, .T. ) ;
#1047=CARTESIAN_POINT ( 'NONE',  ( -4.325729160396026174, -74.16467322009297902, 2.526449232236037901 ) ) ;
#1053=AXIS2_PLACEMENT_3D ( 'NONE', #1447, #1968, #2711 ) ;
#1054=VERTEX_POINT ( 'NONE', #264 ) ;
#1055=CARTESIAN_POINT ( 'NONE',  ( 0.000000000000000000, 0.000000000000000000, 10.00000000000000000 ) ) ;
#1059=CARTESIAN_POINT ( 'NONE',  ( 0.000000000000000000, -80.00000000000000000, 4.999999999999999112 ) ) ;
#1062=CARTESIAN_POINT ( 'NONE',  ( 0.1685493663350521309, 7.499999999999996447, -4.999999999999998224 ) ) ;
#1065=EDGE_LOOP ( 'NONE', ( #1169, #1973 ) ) ;
#1066=CARTESIAN_POINT ( 'NONE',  ( -4.784761898981735762, -50.39152470491934821, 1.451366868840367808 ) ) ;
#1069=DIRECTION ( 'NONE',  ( 0.000000000000000000, 1.000000000000000000, 0.000000000000000000 ) ) ;
#1071=ORIENTED_EDGE ( 'NONE', *, *, #3122, .T. ) ;
#1072=DIRECTION ( 'NONE',  ( 1.000000000000000000, 0.000000000000000000, 0.000000000000000000 ) ) ;
#1073=DIRECTION ( 'NONE',  ( 1.000000000000000000, 0.000000000000000000, 0.000000000000000000 ) ) ;
#1074=CARTESIAN_POINT ( 'NONE',  ( 4.863431995609888148, -5.709553999929329215, 1.172553935287278248 ) ) ;
#1075=CARTESIAN_POINT ( 'NONE',  ( -2.543133226181223616, -7.061565991568797607, 4.317068135836759524 ) ) ;
#1076=EDGE_LOOP ( 'NONE', ( #1151, #2229, #414, #1587, #3090 ) ) ;
#1077=CARTESIAN_POINT ( 'NONE',  ( -0.3416648584763157803, 7.500000000000000888, 5.000000000000000888 ) ) ;
#1079=ORIENTED_EDGE ( 'NONE', *, *, #3194, .T. ) ;
#1084=EDGE_CURVE ( 'NONE', #3146, #3014, #510, .T. ) ;
#1085=CARTESIAN_POINT ( 'NONE',  ( 2.500000000000004441, -71.46446609406727646, 1.464466094067262025 ) ) ;
#1090=CARTESIAN_POINT ( 'NONE',  ( 4.831975997384719612, 5.736714355192817472, -1.328626502536248699 ) ) ;
#1091=CARTESIAN_POINT ( 'NONE',  ( 4.722607672194940598, -5.826754641390677669, 1.650547109183062355 ) ) ;
#1093=VERTEX_POINT ( 'NONE', #1059 ) ;
#1094=CARTESIAN_POINT ( 'NONE',  ( -1.336826802926396995, 7.387368010283515751, -4.829679162932221992 ) ) ;
#1095=AXIS2_PLACEMENT_3D ( 'NONE', #2630, #1582, #841 ) ;
#1101=ORIENTED_EDGE ( 'NONE', *, *, #3177, .F. ) ;
#1102=FACE_OUTER_BOUND ( 'NONE', #1614, .T. ) ;
#1107=( LENGTH_UNIT ( ) NAMED_UNIT ( * ) SI_UNIT ( .MILLI., .METRE. ) );
#1108=CIRCLE ( 'NONE', #2274, 7.500000000000000000 ) ;
#1109=CARTESIAN_POINT ( 'NONE',  ( 4.930411998009738284, 5.651814738127338700, 0.8477781614216437500 ) ) ;
#1110=CARTESIAN_POINT ( 'NONE',  ( 2.500000000000008438, -70.00000000000000000, 10.00000000000000000 ) ) ;
#1111=CARTESIAN_POINT ( 'NONE',  ( -3.320792018548207825, -6.729571896343306214, -3.751470290485135806 ) ) ;
#1114=CARTESIAN_POINT ( 'NONE',  ( -4.725421832813011314, 5.824466512821798503, -1.642406358834817004 ) ) ;
#1115=EDGE_CURVE ( 'NONE', #2713, #1541, #2925, .T. ) ;
#1121=EDGE_LOOP ( 'NONE', ( #833, #2302 ) ) ;
#1129=CARTESIAN_POINT ( 'NONE',  ( 6.124525076959063726E-16, 7.500000000000000000, -4.999999999999999112 ) ) ;
#1130=ADVANCED_FACE ( 'NONE', ( #1524 ), #2535, .T. ) ;
#1132=VERTEX_POINT ( 'NONE', #18 ) ;
#1134=ADVANCED_FACE ( 'NONE', ( #1024 ), #3039, .F. ) ;
#1135=EDGE_LOOP ( 'NONE', ( #2875, #151, #2955, #2834 ) ) ;
#1136=CARTESIAN_POINT ( 'NONE',  ( -2.483052435257200319, -69.66568987240576405, -4.340030773391345242 ) ) ;
#1139=VERTEX_POINT ( 'NONE', #281 ) ;
#1142=CARTESIAN_POINT ( 'NONE',  ( -4.956114419722681852, -5.629162412197389109, 0.6822959203856070465 ) ) ;
#1143=CARTESIAN_POINT ( 'NONE',  ( -4.863431995609888148, 5.709553999929329215, 1.172553935287278248 ) ) ;
#1146=VERTEX_POINT ( 'NONE', #850 ) ;
#1147=EDGE_CURVE ( 'NONE', #97, #1979, #1624, .T. ) ;
#1149=CARTESIAN_POINT ( 'NONE',  ( -5.000000000000001776, -73.31662479035541935, 0.1770536369485815331 ) ) ;
#1151=ORIENTED_EDGE ( 'NONE', *, *, #1928, .F. ) ;
#1153=EDGE_CURVE ( 'NONE', #1895, #84, #746, .T. ) ;
#1155=CARTESIAN_POINT ( 'NONE',  ( 0.000000000000000000, -60.00000000000000000, -2.500000000000000444 ) ) ;
#1159=AXIS2_PLACEMENT_3D ( 'NONE', #650, #2663, #143 ) ;
#1164=( GEOMETRIC_REPRESENTATION_CONTEXT ( 3 ) GLOBAL_UNCERTAINTY_ASSIGNED_CONTEXT ( ( #1792 ) ) GLOBAL_UNIT_ASSIGNED_CONTEXT ( ( #1945, #2710, #3216 ) ) REPRESENTATION_CONTEXT ( 'NONE', 'WORKASPACE' ) );
#1165=ORIENTED_EDGE ( 'NONE', *, *, #942, .F. ) ;
#1167=CARTESIAN_POINT ( 'NONE',  ( 2.417876621355959710, -70.65655750441386829, -4.376674006154569696 ) ) ;
#1168=CARTESIAN_POINT ( 'NONE',  ( 6.121942914840092871E-16, -7.500000000000000000, -4.999999999999999112 ) ) ;
#1169=ORIENTED_EDGE ( 'NONE', *, *, #1285, .T. ) ;
#1170=FACE_OUTER_BOUND ( 'NONE', #1076, .T. ) ;
#1172=CARTESIAN_POINT ( 'NONE',  ( 2.243056629538943803, -68.88414527589007719, -4.469195550069930967 ) ) ;
#1173=CARTESIAN_POINT ( 'NONE',  ( 3.984264206898686211, -74.49240233626514396, 3.036427941355731797 ) ) ;
#1174=CARTESIAN_POINT ( 'NONE',  ( -4.985720285031673527, -48.54819230487149895, -0.3898302721915644087 ) ) ;
#1177=CARTESIAN_POINT ( 'NONE',  ( 3.061616997868384127E-16, -67.50000000000000000, 2.500000000000000444 ) ) ;
#1182=DIRECTION ( 'NONE',  ( 0.000000000000000000, 1.000000000000000000, 0.000000000000000000 ) ) ;
#1185=CARTESIAN_POINT ( 'NONE',  ( 2.592701047953016147, -64.58086786481547392, 4.287209529367743244 ) ) ;
#1186=LINE ( 'NONE', #2715, #1939 ) ;
#1187=CARTESIAN_POINT ( 'NONE',  ( 1.464466094067263358, -67.50000000000000000, -2.500000000000002220 ) ) ;
#1188=CARTESIAN_POINT ( 'NONE',  ( 0.3480864936855372904, -75.99245047245101148, 4.990948402655850380 ) ) ;
#1190=CARTESIAN_POINT ( 'NONE',  ( -4.815134987083422580, -49.33398324077673180, 1.347591700989805741 ) ) ;
#1192=CARTESIAN_POINT ( 'NONE',  ( 4.815279722017292485, -49.33289952491914931, -1.347079874192880444 ) ) ;
#1195=VERTEX_POINT ( 'NONE', #557 ) ;
#1198=LINE ( 'NONE', #931, #2596 ) ;
#1199=DIRECTION ( 'NONE',  ( 1.000000000000000000, 0.000000000000000000, 0.000000000000000000 ) ) ;
#1201=CARTESIAN_POINT ( 'NONE',  ( 3.117741096646119203, -64.86494573768398197, 3.921983519476098135 ) ) ;
#1203=DIRECTION ( 'NONE',  ( 0.000000000000000000, 1.000000000000000000, 0.000000000000000000 ) ) ;
#1209=CYLINDRICAL_SURFACE ( 'NONE', #86, 4.999999999999999112 ) ;
#1211=ORIENTED_EDGE ( 'NONE', *, *, #411, .T. ) ;
#1214=DIRECTION ( 'NONE',  ( 0.000000000000000000, 0.000000000000000000, -1.000000000000000000 ) ) ;
#1215=VECTOR ( 'NONE', #788, 1000.000000000000000 ) ;
#1216=CYLINDRICAL_SURFACE ( 'NONE', #2435, 2.499999999999999556 ) ;
#1217=B_SPLINE_CURVE_WITH_KNOTS ( 'NONE', 3,
 ( #284, #21, #1560, #3042, #2826, #2566, #1042, #574, #754, #301, #1509, #1310, #4, #268, #1258, #319, #51, #1327, #1013, #34, #2043, #785, #2028, #249, #2293, #1028, #1787, #2796 ),
 .UNSPECIFIED., .F., .F.,
 ( 4, 2, 2, 2, 2, 2, 2, 2, 2, 2, 2, 2, 2, 4 ),
 ( 0.004716923349278730540, 0.005306377133062306975, 0.005601104024954096060, 0.005895830916845884277, 0.006485284700629445967, 0.006780011592521222909, 0.007074738484412999850, 0.007369465376304777660, 0.007664192268196553734, 0.008253646051980109352, 0.008548372943871894100, 0.008843099835763678848, 0.009137826727655463596, 0.009432553619547248344 ),
 .UNSPECIFIED. ) ;
#1218=DIRECTION ( 'NONE',  ( 1.000000000000000000, 0.000000000000000000, 0.000000000000000000 ) ) ;
#1222=CARTESIAN_POINT ( 'NONE',  ( 4.962858103399386600, -73.37410943649805972, 0.6966535907275263062 ) ) ;
#1223=CARTESIAN_POINT ( 'NONE',  ( 0.000000000000000000, -72.50000000000001421, -2.500000000000000444 ) ) ;
#1230=EDGE_CURVE ( 'NONE', #2520, #2101, #1217, .T. ) ;
#1231=CARTESIAN_POINT ( 'NONE',  ( 4.481108542057384625, -6.016226048536217341, -2.241414944841849888 ) ) ;
#1232=CYLINDRICAL_SURFACE ( 'NONE', #794, 2.500000000000000444 ) ;
#1235=ORIENTED_EDGE ( 'NONE', *, *, #2947, .F. ) ;
#1240=DIRECTION ( 'NONE',  ( 0.000000000000000000, 0.000000000000000000, 1.000000000000000000 ) ) ;
#1245=CARTESIAN_POINT ( 'NONE',  ( -3.117018002318639347, -64.86457393883293321, 3.922457828541068281 ) ) ;
#1246=AXIS2_PLACEMENT_3D ( 'NONE', #3052, #43, #1749 ) ;
#1247=CARTESIAN_POINT ( 'NONE',  ( 4.716912583111714241, -66.29091800361955222, 1.666493794562607711 ) ) ;
#1249=CARTESIAN_POINT ( 'NONE',  ( 0.000000000000000000, -80.00000000000000000, 0.000000000000000000 ) ) ;
#1258=CARTESIAN_POINT ( 'NONE',  ( 4.997074555615626856, -51.49033316323540532, -0.1965204501117691904 ) ) ;
#1259=CARTESIAN_POINT ( 'NONE',  ( 3.320170879781855433, -6.729821324027721374, 3.751849819826997834 ) ) ;
#1261=CARTESIAN_POINT ( 'NONE',  ( -4.871060595381011993, -50.99085979125018753, 1.130390421582378124 ) ) ;
#1264=FACE_OUTER_BOUND ( 'NONE', #3204, .T. ) ;
#1269=ORIENTED_EDGE ( 'NONE', *, *, #2510, .T. ) ;
#1271=CARTESIAN_POINT ( 'NONE',  ( 1.181079518071022826E-19, -64.00000000000000000, 4.999999999999999112 ) ) ;
#1273=DIRECTION ( 'NONE',  ( 0.000000000000000000, 0.000000000000000000, 1.000000000000000000 ) ) ;
#1274=DIRECTION ( 'NONE',  ( 0.000000000000000000, 1.000000000000000000, 0.000000000000000000 ) ) ;
#1278=CARTESIAN_POINT ( 'NONE',  ( -3.791988745706118102, -65.34238691411069055, 3.273615902745505846 ) ) ;
#1279=CARTESIAN_POINT ( 'NONE',  ( -4.916101592540525367, -51.19835914624871975, -0.9229043554563169938 ) ) ;
#1281=DIRECTION ( 'NONE',  ( -0.000000000000000000, -1.000000000000000000, -0.000000000000000000 ) ) ;
#1285=EDGE_CURVE ( 'NONE', #1384, #1132, #1725, .T. ) ;
#1287=CARTESIAN_POINT ( 'NONE',  ( 8.572527594031472993E-15, -70.00000000000000000, 0.000000000000000000 ) ) ;
#1288=CARTESIAN_POINT ( 'NONE',  ( -3.321910197521175778, -6.728960966335735705, 3.750313380908745664 ) ) ;
#1289=EDGE_CURVE ( 'NONE', #1132, #721, #1291, .T. ) ;
#1291=LINE ( 'NONE', #2306, #775 ) ;
#1295=CARTESIAN_POINT ( 'NONE',  ( -3.359134405502826048, -74.97878567386173643, 3.716361166143389294 ) ) ;
#1300=FACE_OUTER_BOUND ( 'NONE', #1135, .T. ) ;
#1305=PRESENTATION_STYLE_ASSIGNMENT (( #3112 ) ) ;
#1308=LINE ( 'NONE', #299, #2827 ) ;
#1310=CARTESIAN_POINT ( 'NONE',  ( 4.996981400519024952, -51.49002086460089345, 0.1986267936440539450 ) ) ;
#1314=CARTESIAN_POINT ( 'NONE',  ( -4.927416625552392127, -73.42405444405065396, 0.8653657731671230424 ) ) ;
#1317=DIRECTION ( 'NONE',  ( -1.000000000000000000, 0.000000000000000000, 0.000000000000000000 ) ) ;
#1319=VECTOR ( 'NONE', #2742, 1000.000000000000000 ) ;
#1326=ORIENTED_EDGE ( 'NONE', *, *, #2132, .T. ) ;
#1327=CARTESIAN_POINT ( 'NONE',  ( 4.945771905224659371, -51.30991108704697012, -0.7565992915569080823 ) ) ;
#1329=ORIENTED_EDGE ( 'NONE', *, *, #1029, .T. ) ;
#1334=CARTESIAN_POINT ( 'NONE',  ( 6.123233995736765296E-16, -80.00000000000000000, -4.999999999999999112 ) ) ;
#1337=CYLINDRICAL_SURFACE ( 'NONE', #3067, 2.499999999999999556 ) ;
#1338=CARTESIAN_POINT ( 'NONE',  ( 4.999850703040199740, 5.590303478919644853, 0.1739517833579089512 ) ) ;
#1339=CARTESIAN_POINT ( 'NONE',  ( 1.181079518071022826E-19, -64.00000000000000000, 4.999999999999999112 ) ) ;
#1341=ORIENTED_EDGE ( 'NONE', *, *, #1643, .T. ) ;
#1342=CARTESIAN_POINT ( 'NONE',  ( -3.772047191027663615, 6.487346954507292374, -3.297239103104800506 ) ) ;
#1346=ORIENTED_EDGE ( 'NONE', *, *, #473, .T. ) ;
#1347=CARTESIAN_POINT ( 'NONE',  ( 4.999999999999999112, -66.68337520964459486, 0.000000000000000000 ) ) ;
#1350=( NAMED_UNIT ( * ) PLANE_ANGLE_UNIT ( ) SI_UNIT ( $, .RADIAN. ) );
#1353=ORIENTED_EDGE ( 'NONE', *, *, #1965, .T. ) ;
#1355=FACE_OUTER_BOUND ( 'NONE', #183, .T. ) ;
#1357=CARTESIAN_POINT ( 'NONE',  ( 3.077296587540346184, 6.845542784947758364, -3.953776968828220717 ) ) ;
#1358=CARTESIAN_POINT ( 'NONE',  ( -4.962858103399387488, -66.62589056350195449, 0.6966535907275258621 ) ) ;
#1359=CARTESIAN_POINT ( 'NONE',  ( -4.990888858476322021, -5.598354044414833197, 0.3458703032855571791 ) ) ;
#1364=( BOUNDED_CURVE ( )  B_SPLINE_CURVE ( 3, ( #2220, #1187, #2959, #2483 ),
 .UNSPECIFIED., .F., .T. ) 
 B_SPLINE_CURVE_WITH_KNOTS ( ( 4, 4 ),
 ( 3.141592653589791340, 4.712388980384689674 ),
 .UNSPECIFIED. ) 
 CURVE ( )  GEOMETRIC_REPRESENTATION_ITEM ( )  RATIONAL_B_SPLINE_CURVE ( ( 1.000000000000000000, 0.8047378541243646044, 0.8047378541243646044, 1.000000000000000000 ) ) 
 REPRESENTATION_ITEM ( '' )  );
#1365=CARTESIAN_POINT ( 'NONE',  ( -4.999999999999999112, -73.31662479035540514, 0.000000000000000000 ) ) ;
#1368=DIRECTION ( 'NONE',  ( 0.000000000000000000, 0.000000000000000000, 1.000000000000000000 ) ) ;
#1372=CIRCLE ( 'NONE', #2168, 4.999999999999999112 ) ;
#1373=ADVANCED_FACE ( 'NONE', ( #2093 ), #85, .F. ) ;
#1374=DIRECTION ( 'NONE',  ( -1.000000000000000000, 0.000000000000000000, 0.000000000000000000 ) ) ;
#1376=CARTESIAN_POINT ( 'NONE',  ( 0.000000000000000000, 7.500000000000000000, 4.999999999999999112 ) ) ;
#1380=CARTESIAN_POINT ( 'NONE',  ( -0.3368283383274193743, 7.494339828221662003, -4.991522157455978714 ) ) ;
#1383=CARTESIAN_POINT ( 'NONE',  ( 0.000000000000000000, 80.00000000000000000, 0.000000000000000000 ) ) ;
#1384=VERTEX_POINT ( 'NONE', #2130 ) ;
#1386=CARTESIAN_POINT ( 'NONE',  ( 4.999999999999999112, -80.00000000000000000, 0.000000000000000000 ) ) ;
#1387=CARTESIAN_POINT ( 'NONE',  ( 0.3332490247102218861, -67.51676079561944732, -4.991558521926720005 ) ) ;
#1389=CARTESIAN_POINT ( 'NONE',  ( 2.500000000000004441, -70.00000000000000000, 0.000000000000000000 ) ) ;
#1396=EDGE_CURVE ( 'NONE', #84, #1895, #1536, .T. ) ;
#1402=CARTESIAN_POINT ( 'NONE',  ( 0.000000000000000000, 0.000000000000000000, -10.00000000000000000 ) ) ;
#1405=CARTESIAN_POINT ( 'NONE',  ( -1.464466094067257806, -72.50000000000001421, 2.499999999999999556 ) ) ;
#1420=CARTESIAN_POINT ( 'NONE',  ( 6.122861072698252249E-16, -67.50000000000000000, -4.999999999999999112 ) ) ;
#1421=ORIENTED_EDGE ( 'NONE', *, *, #1153, .T. ) ;
#1422=DIRECTION ( 'NONE',  ( 0.000000000000000000, 0.000000000000000000, 1.000000000000000000 ) ) ;
#1425=CARTESIAN_POINT ( 'NONE',  ( -0.8424979979451828749, -7.454395415945072045, -4.931395878866434046 ) ) ;
#1432=CARTESIAN_POINT ( 'NONE',  ( 8.572527594031472993E-15, -70.00000000000000000, 10.00000000000000000 ) ) ;
#1434=CARTESIAN_POINT ( 'NONE',  ( 4.954123618475600566, -66.61507573143732941, 0.6974948150963297122 ) ) ;
#1439=CARTESIAN_POINT ( 'NONE',  ( -4.815309899926791815, -49.33271645601669775, -1.346969744587360074 ) ) ;
#1447=CARTESIAN_POINT ( 'NONE',  ( 0.000000000000000000, 0.000000000000000000, -10.00000000000000000 ) ) ;
#1448=ORIENTED_EDGE ( 'NONE', *, *, #983, .T. ) ;
#1456=FACE_BOUND ( 'NONE', #2903, .T. ) ;
#1459=ORIENTED_EDGE ( 'NONE', *, *, #2588, .T. ) ;
#1461=CIRCLE ( 'NONE', #2207, 2.500000000000000000 ) ;
#1462=CARTESIAN_POINT ( 'NONE',  ( 0.6557238592495003848, -72.41814643914202065, -4.959498321622188399 ) ) ;
#1463=CARTESIAN_POINT ( 'NONE',  ( 0.1683266833682984520, -7.500000000000003553, -5.000000000000000000 ) ) ;
#1466=CARTESIAN_POINT ( 'NONE',  ( 4.999999999999999112, -66.68337520964459486, 0.000000000000000000 ) ) ;
#1467=CIRCLE ( 'NONE', #3267, 6.000000000000001776 ) ;
#1473=CARTESIAN_POINT ( 'NONE',  ( 4.856148773929144902, -49.08427523399102910, 1.192039989181127080 ) ) ;
#1478=ORIENTED_EDGE ( 'NONE', *, *, #1147, .F. ) ;
#1481=AXIS2_PLACEMENT_3D ( 'NONE', #1679, #2953, #693 ) ;
#1487=B_SPLINE_CURVE_WITH_KNOTS ( 'NONE', 3,
 ( #188, #173, #1932, #3205, #1697, #2218, #1681, #2461, #1185, #1201, #1500, #1711, #428, #3221, #1728, #2509, #1247, #679, #2696, #2714, #1434, #2200, #1950, #1466 ),
 .UNSPECIFIED., .F., .F.,
 ( 4, 2, 2, 2, 2, 2, 2, 2, 2, 2, 2, 4 ),
 ( 0.008369288751650572414, 0.008891570837864926427, 0.009413852924079280440, 0.01045841709650799541, 0.01150298126893671211, 0.01254754544136542707, 0.01359210961379414551, 0.01463667378622286047, 0.01515895587243720928, 0.01568123795865155809, 0.01620352004486590863, 0.01672580213108025918 ),
 .UNSPECIFIED. ) ;
#1497=EDGE_LOOP ( 'NONE', ( #2982, #1646, #2810, #187, #3136, #645, #1781 ) ) ;
#1499=CARTESIAN_POINT ( 'NONE',  ( 0.000000000000000000, -7.500000000000000000, 4.999999999999999112 ) ) ;
#1500=CARTESIAN_POINT ( 'NONE',  ( 3.359134405502826048, -65.02121432613829199, 3.716361166143391959 ) ) ;
#1504=DIRECTION ( 'NONE',  ( 0.000000000000000000, 0.000000000000000000, 1.000000000000000000 ) ) ;
#1506=CARTESIAN_POINT ( 'NONE',  ( 4.977308113077120844, -48.57700265276938012, 0.4845947803478808380 ) ) ;
#1509=CARTESIAN_POINT ( 'NONE',  ( 4.985625624127048461, -51.45148266395612069, 0.3909128500499727821 ) ) ;
#1510=CARTESIAN_POINT ( 'NONE',  ( 3.766216509439173965, -6.490735160851770047, 3.303865152441167297 ) ) ;
#1511=VECTOR ( 'NONE', #2371, 1000.000000000000000 ) ;
#1512=ADVANCED_FACE ( 'NONE', ( #1456, #197 ), #1209, .T. ) ;
#1513=CARTESIAN_POINT ( 'NONE',  ( -4.772823807329270807, -50.19767535498903754, -1.490153625805560322 ) ) ;
#1515=FACE_BOUND ( 'NONE', #1065, .T. ) ;
#1516=VECTOR ( 'NONE', #272, 1000.000000000000000 ) ;
#1517=EDGE_CURVE ( 'NONE', #2753, #1195, #764, .T. ) ;
#1518=B_SPLINE_CURVE_WITH_KNOTS ( 'NONE', 3,
 ( #2920, #2118, #1136, #3127, #598, #2416, #2677, #2871, #2648, #2167, #3176, #904, #648, #94, #2616, #861, #1915, #361 ),
 .UNSPECIFIED., .F., .F.,
 ( 4, 2, 2, 2, 2, 2, 2, 2, 4 ),
 ( 0.007951492273476376202, 0.008447850770476991039, 0.008944209267477605876, 0.009440567764478220714, 0.009936926261478833816, 0.01043328475847945039, 0.01092964325548006349, 0.01142600175248067833, 0.01192236024948129317 ),
 .UNSPECIFIED. ) ;
#1519=DIRECTION ( 'NONE',  ( 0.000000000000000000, 0.000000000000000000, -1.000000000000000000 ) ) ;
#1520=AXIS2_PLACEMENT_3D ( 'NONE', #3260, #2252, #512 ) ;
#1523=CARTESIAN_POINT ( 'NONE',  ( 2.368532205790481182, -70.81652027702884311, -4.403989053656482966 ) ) ;
#1524=FACE_OUTER_BOUND ( 'NONE', #597, .T. ) ;
#1527=CARTESIAN_POINT ( 'NONE',  ( 0.6733179620838674051, 7.471617105689219329, -4.957340513892267708 ) ) ;
#1528=CARTESIAN_POINT ( 'NONE',  ( 4.324630367402185982, -6.131366064188266130, 2.529815037953009327 ) ) ;
#1530=CARTESIAN_POINT ( 'NONE',  ( -1.181079518071022826E-19, -76.00000000000001421, 4.999999999999999112 ) ) ;
#1532=AXIS2_PLACEMENT_3D ( 'NONE', #3270, #2029, #2372 ) ;
#1535=CARTESIAN_POINT ( 'NONE',  ( 0.000000000000000000, -60.00000000000000000, -2.500000000000000444 ) ) ;
#1536=B_SPLINE_CURVE_WITH_KNOTS ( 'NONE', 3,
 ( #1129, #1628, #1380, #2144, #2110, #1094, #625, #607, #2671, #1594, #2641, #1342, #2375, #103, #641, #3117, #1114, #871, #2897, #1837, #1872, #387, #133, #1143, #3151, #2609, #2845, #336, #2160, #370, #400, #2341, #591, #2395, #2357, #1642, #2656, #68, #1077, #3184 ),
 .UNSPECIFIED., .F., .F.,
 ( 4, 2, 2, 2, 2, 2, 2, 2, 2, 2, 2, 2, 2, 2, 2, 2, 2, 2, 2, 4 ),
 ( 0.01615986362459447684, 0.01666419217584455895, 0.01716852072709463758, 0.01817717782959479833, 0.01918583493209496255, 0.02019449203459512329, 0.02120314913709528404, 0.02221180623959544478, 0.02271613479084552342, 0.02322046334209560553, 0.02422912044459576628, 0.02523777754709592702, 0.02574210609834600566, 0.02624643464959608777, 0.02725509175209624851, 0.02826374885459641273, 0.02927240595709657001, 0.03028106305959672728, 0.03128972016209689150, 0.03229837726459704877 ),
 .UNSPECIFIED. ) ;
#1541=VERTEX_POINT ( 'NONE', #3264 ) ;
#1542=FACE_OUTER_BOUND ( 'NONE', #2880, .T. ) ;
#1543=( NAMED_UNIT ( * ) PLANE_ANGLE_UNIT ( ) SI_UNIT ( $, .RADIAN. ) );
#1545=CARTESIAN_POINT ( 'NONE',  ( -1.654849718955805127, -7.321828482412975347, 4.729586325473386310 ) ) ;
#1546=ORIENTED_EDGE ( 'NONE', *, *, #1517, .F. ) ;
#1547=DIRECTION ( 'NONE',  ( -1.000000000000000000, 0.000000000000000000, 0.000000000000000000 ) ) ;
#1550=CARTESIAN_POINT ( 'NONE',  ( -4.769696007084729850, -50.00000000000000000, 1.499999999999994449 ) ) ;
#1560=CARTESIAN_POINT ( 'NONE',  ( 4.782644271597511043, -50.39484142078823226, 1.460283231774381907 ) ) ;
#1562=CARTESIAN_POINT ( 'NONE',  ( -4.716912583111715129, -73.70908199638046199, 1.666493794562607933 ) ) ;
#1563=CARTESIAN_POINT ( 'NONE',  ( 0.000000000000000000, -60.00000000000000000, 0.000000000000000000 ) ) ;
#1569=VERTEX_POINT ( 'NONE', #2070 ) ;
#1573=ADVANCED_FACE ( 'NONE', ( #515, #1542 ), #1767, .T. ) ;
#1575=CARTESIAN_POINT ( 'NONE',  ( 0.000000000000000000, -72.50000000000001421, -2.500000000000000444 ) ) ;
#1576=EDGE_LOOP ( 'NONE', ( #2037, #1632, #2864, #260, #1799, #1604 ) ) ;
#1577=CARTESIAN_POINT ( 'NONE',  ( 0.8424979979451828749, 7.454395415945072045, -4.931395878866434046 ) ) ;
#1580=CARTESIAN_POINT ( 'NONE',  ( -4.987611521976591078, -51.45995144009268074, -0.3958319429405975920 ) ) ;
#1581=VECTOR ( 'NONE', #920, 1000.000000000000000 ) ;
#1582=DIRECTION ( 'NONE',  ( -0.000000000000000000, -0.000000000000000000, -1.000000000000000000 ) ) ;
#1584=CARTESIAN_POINT ( 'NONE',  ( 0.000000000000000000, 0.000000000000000000, -10.00000000000000000 ) ) ;
#1587=ORIENTED_EDGE ( 'NONE', *, *, #2588, .F. ) ;
#1588=DIRECTION ( 'NONE',  ( 1.000000000000000000, 0.000000000000000000, 0.000000000000000000 ) ) ;
#1590=CARTESIAN_POINT ( 'NONE',  ( 5.000292928619530564, 5.589907940605836956, -0.3348667354298545673 ) ) ;
#1591=CARTESIAN_POINT ( 'NONE',  ( -2.312079649032890760, -64.45380699776846711, 4.445949067509105568 ) ) ;
#1592=CARTESIAN_POINT ( 'NONE',  ( -3.078112602769041306, -6.845324219060942461, 3.953457562721318652 ) ) ;
#1594=CARTESIAN_POINT ( 'NONE',  ( -3.078327448814686562, 6.845130131842670274, -3.953084837412474517 ) ) ;
#1597=ORIENTED_EDGE ( 'NONE', *, *, #755, .T. ) ;
#1598=CARTESIAN_POINT ( 'NONE',  ( -1.532095834638425913, -71.98215106548155973, -4.761538506183794262 ) ) ;
#1600=ORIENTED_EDGE ( 'NONE', *, *, #672, .T. ) ;
#1604=ORIENTED_EDGE ( 'NONE', *, *, #1115, .F. ) ;
#1605=CYLINDRICAL_SURFACE ( 'NONE', #740, 6.000000000000001776 ) ;
#1607=CARTESIAN_POINT ( 'NONE',  ( 3.320792018548207825, 6.729571896343306214, -3.751470290485135806 ) ) ;
#1614=EDGE_LOOP ( 'NONE', ( #2024, #2244, #3174, #3066, #2457 ) ) ;
#1620=LINE ( 'NONE', #1652, #1581 ) ;
#1623=DIRECTION ( 'NONE',  ( -0.000000000000000000, -0.000000000000000000, -1.000000000000000000 ) ) ;
#1624=LINE ( 'NONE', #2623, #1511 ) ;
#1627=EDGE_LOOP ( 'NONE', ( #373, #3027 ) ) ;
#1628=CARTESIAN_POINT ( 'NONE',  ( -0.1683266833682984520, 7.500000000000003553, -5.000000000000000000 ) ) ;
#1630=VERTEX_POINT ( 'NONE', #1021 ) ;
#1631=DIRECTION ( 'NONE',  ( 0.000000000000000000, 1.000000000000000000, 0.000000000000000000 ) ) ;
#1632=ORIENTED_EDGE ( 'NONE', *, *, #2617, .T. ) ;
#1633=CYLINDRICAL_SURFACE ( 'NONE', #2702, 2.499999999999999556 ) ;
#1634=LINE ( 'NONE', #344, #980 ) ;
#1635=FACE_OUTER_BOUND ( 'NONE', #1674, .T. ) ;
#1636=APPLICATION_CONTEXT ( 'automotive_design' ) ;
#1637=ORIENTED_EDGE ( 'NONE', *, *, #2448, .T. ) ;
#1641=CARTESIAN_POINT ( 'NONE',  ( -0.1685493663350521309, -7.499999999999996447, -4.999999999999998224 ) ) ;
#1642=CARTESIAN_POINT ( 'NONE',  ( -1.658007454526697177, 7.321065759480116952, 4.728400501374060205 ) ) ;
#1643=EDGE_CURVE ( 'NONE', #1569, #3146, #829, .T. ) ;
#1646=ORIENTED_EDGE ( 'NONE', *, *, #986, .T. ) ;
#1647=CARTESIAN_POINT ( 'NONE',  ( -2.499999999999990230, -70.16572065136264769, -4.330127018922198090 ) ) ;
#1648=PRODUCT_DEFINITION ( 'UNKNOWN', '', #1849, #506 ) ;
#1649=ORIENTED_EDGE ( 'NONE', *, *, #1789, .T. ) ;
#1652=CARTESIAN_POINT ( 'NONE',  ( 7.500000000000000000, 9.184850993605147944E-16, 10.00000000000000000 ) ) ;
#1661=CYLINDRICAL_SURFACE ( 'NONE', #1481, 2.500000000000000444 ) ;
#1662=ORIENTED_EDGE ( 'NONE', *, *, #1043, .T. ) ;
#1663=CYLINDRICAL_SURFACE ( 'NONE', #947, 4.999999999999999112 ) ;
#1667=CARTESIAN_POINT ( 'NONE',  ( -4.769696007084729850, -50.00000000000000000, 1.499999999999994449 ) ) ;
#1674=EDGE_LOOP ( 'NONE', ( #1706, #2788 ) ) ;
#1677=EDGE_CURVE ( 'NONE', #1911, #2713, #2948, .T. ) ;
#1678=CIRCLE ( 'NONE', #1729, 6.000000000000001776 ) ;
#1679=CARTESIAN_POINT ( 'NONE',  ( 0.000000000000000000, -60.00000000000000000, 0.000000000000000000 ) ) ;
#1680=ORIENTED_EDGE ( 'NONE', *, *, #2510, .F. ) ;
#1681=CARTESIAN_POINT ( 'NONE',  ( 1.696011499264681532, -64.23548717087807347, 4.715485471644023541 ) ) ;
#1692=AXIS2_PLACEMENT_3D ( 'NONE', #3075, #2051, #2104 ) ;
#1693=ORIENTED_EDGE ( 'NONE', *, *, #1928, .T. ) ;
#1697=CARTESIAN_POINT ( 'NONE',  ( 0.8675805444301170066, -64.06058600797459235, 4.927173720332874041 ) ) ;
#1698=LINE ( 'NONE', #935, #2155 ) ;
#1701=FACE_OUTER_BOUND ( 'NONE', #389, .T. ) ;
#1703=CARTESIAN_POINT ( 'NONE',  ( 2.500000000000008438, -70.00000000000000000, 10.00000000000000000 ) ) ;
#1706=ORIENTED_EDGE ( 'NONE', *, *, #2414, .F. ) ;
#1709=CARTESIAN_POINT ( 'NONE',  ( 0.6741883319902871596, -7.471549563736964217, -4.957238835368188212 ) ) ;
#1710=ORIENTED_EDGE ( 'NONE', *, *, #2762, .F. ) ;
#1711=CARTESIAN_POINT ( 'NONE',  ( 3.790413940515792390, -65.34115326502070786, 3.275345238443577944 ) ) ;
#1715=ADVANCED_FACE ( 'NONE', ( #1355 ), #866, .T. ) ;
#1716=ORIENTED_EDGE ( 'NONE', *, *, #2762, .T. ) ;
#1718=EDGE_CURVE ( 'NONE', #1630, #1979, #2277, .T. ) ;
#1723=ORIENTED_EDGE ( 'NONE', *, *, #1153, .F. ) ;
#1725=CIRCLE ( 'NONE', #296, 2.499999999999999556 ) ;
#1727=DIRECTION ( 'NONE',  ( 0.000000000000000000, 0.000000000000000000, 1.000000000000000000 ) ) ;
#1728=CARTESIAN_POINT ( 'NONE',  ( 4.475554532957461085, -65.99917996832718359, 2.251442214368883477 ) ) ;
#1729=AXIS2_PLACEMENT_3D ( 'NONE', #240, #1504, #2528 ) ;
#1732=ORIENTED_EDGE ( 'NONE', *, *, #59, .T. ) ;
#1739=ADVANCED_FACE ( 'NONE', ( #2405 ), #1337, .F. ) ;
#1743=AXIS2_PLACEMENT_3D ( 'NONE', #331, #2351, #1832 ) ;
#1745=CARTESIAN_POINT ( 'NONE',  ( 0.3416648584763157803, -7.500000000000000888, 5.000000000000000888 ) ) ;
#1746=FACE_OUTER_BOUND ( 'NONE', #1121, .T. ) ;
#1748=VERTEX_POINT ( 'NONE', #1389 ) ;
#1749=DIRECTION ( 'NONE',  ( 0.000000000000000000, 0.000000000000000000, -1.000000000000000000 ) ) ;
#1751=CARTESIAN_POINT ( 'NONE',  ( 4.856127559802944305, -49.08436397556629061, -1.192133730937313008 ) ) ;
#1758=EDGE_CURVE ( 'NONE', #1093, #129, #3131, .T. ) ;
#1762=CYLINDRICAL_SURFACE ( 'NONE', #2539, 2.499999999999999556 ) ;
#1766=ORIENTED_EDGE ( 'NONE', *, *, #2947, .T. ) ;
#1767=CYLINDRICAL_SURFACE ( 'NONE', #2830, 7.500000000000000000 ) ;
#1770=CARTESIAN_POINT ( 'NONE',  ( 1.654328459400600471, 7.322002074975777930, -4.729864656991090932 ) ) ;
#1772=CARTESIAN_POINT ( 'NONE',  ( -4.724063086364457931, -66.29587799920766145, 1.668329630282862963 ) ) ;
#1773=CIRCLE ( 'NONE', #2885, 7.500000000000000000 ) ;
#1774=CARTESIAN_POINT ( 'NONE',  ( -4.769696007084725409, -50.09973230823852219, -1.500000000000006661 ) ) ;
#1776=DIRECTION ( 'NONE',  ( -1.000000000000000000, 0.000000000000000000, 0.000000000000000000 ) ) ;
#1778=EDGE_CURVE ( 'NONE', #842, #216, #690, .T. ) ;
#1781=ORIENTED_EDGE ( 'NONE', *, *, #401, .F. ) ;
#1782=DIRECTION ( 'NONE',  ( 0.000000000000000000, 1.000000000000000000, 0.000000000000000000 ) ) ;
#1783=CARTESIAN_POINT ( 'NONE',  ( 2.500000000000008438, -70.00000000000000000, -4.330127018922187432 ) ) ;
#1787=CARTESIAN_POINT ( 'NONE',  ( 4.769696007084725409, -50.09970496801165751, -1.500000000000006217 ) ) ;
#1789=EDGE_CURVE ( 'NONE', #2919, #2109, #2645, .T. ) ;
#1791=CARTESIAN_POINT ( 'NONE',  ( -0.8675805444301208924, -75.93941399202543607, 4.927173720332874041 ) ) ;
#1792=UNCERTAINTY_MEASURE_WITH_UNIT (LENGTH_MEASURE( 1.000000000000000082E-05 ), #1945, 'distance_accuracy_value', 'NONE');
#1795=CYLINDRICAL_SURFACE ( 'NONE', #2780, 7.500000000000000000 ) ;
#1799=ORIENTED_EDGE ( 'NONE', *, *, #2087, .F. ) ;
#1808=CARTESIAN_POINT ( 'NONE',  ( -4.997016223860688555, -51.49013799948261294, 0.1978941090189494934 ) ) ;
#1815=DIRECTION ( 'NONE',  ( -0.000000000000000000, -0.000000000000000000, -1.000000000000000000 ) ) ;
#1819=ORIENTED_EDGE ( 'NONE', *, *, #811, .T. ) ;
#1821=ADVANCED_FACE ( 'NONE', ( #2860 ), #1605, .T. ) ;
#1824=CARTESIAN_POINT ( 'NONE',  ( -4.784663389310397363, -50.39016944930146735, -1.451689076663209566 ) ) ;
#1832=DIRECTION ( 'NONE',  ( 0.000000000000000000, 0.000000000000000000, -1.000000000000000000 ) ) ;
#1833=CARTESIAN_POINT ( 'NONE',  ( -1.464466094067260249, -67.50000000000000000, -2.499999999999996447 ) ) ;
#1834=CARTESIAN_POINT ( 'NONE',  ( 3.966867482980610315, -6.368676471623262003, 3.060450018115215443 ) ) ;
#1837=CARTESIAN_POINT ( 'NONE',  ( -4.965855707945498132, 5.621220898751191797, -0.6727113530297602617 ) ) ;
#1840=CARTESIAN_POINT ( 'NONE',  ( -1.263489017627365207, -72.16329285933299786, -4.839748143728395569 ) ) ;
#1842=ORIENTED_EDGE ( 'NONE', *, *, #1029, .F. ) ;
#1843=FACE_BOUND ( 'NONE', #29, .T. ) ;
#1844=CARTESIAN_POINT ( 'NONE',  ( 0.000000000000000000, -60.00000000000000000, 0.000000000000000000 ) ) ;
#1846=ORIENTED_EDGE ( 'NONE', *, *, #1396, .T. ) ;
#1849=PRODUCT_DEFINITION_FORMATION_WITH_SPECIFIED_SOURCE ( 'ANY', '', #2159, .NOT_KNOWN. ) ;
#1850=CARTESIAN_POINT ( 'NONE',  ( 4.325873777034227707, 6.130418473463322471, -2.527359400829327196 ) ) ;
#1851=DIRECTION ( 'NONE',  ( -0.000000000000000000, -0.000000000000000000, 1.000000000000000000 ) ) ;
#1852=LINE ( 'NONE', #814, #466 ) ;
#1854=DIRECTION ( 'NONE',  ( -0.000000000000000000, -0.000000000000000000, 1.000000000000000000 ) ) ;
#1856=ORIENTED_EDGE ( 'NONE', *, *, #1043, .F. ) ;
#1861=DIRECTION ( 'NONE',  ( 0.000000000000000000, 1.000000000000000000, 0.000000000000000000 ) ) ;
#1863=CARTESIAN_POINT ( 'NONE',  ( 2.500000000000008438, -69.83207023104499456, -4.330127018922187432 ) ) ;
#1868=CARTESIAN_POINT ( 'NONE',  ( 0.6766787981060014001, 7.476722154948000743, 4.965272001127371659 ) ) ;
#1870=CARTESIAN_POINT ( 'NONE',  ( -4.966432541228214426, -5.620714496023337503, -0.6691698110145376521 ) ) ;
#1871=EDGE_LOOP ( 'NONE', ( #3062, #1326, #2154, #421, #1662, #3162, #2579, #1346, #1546, #2340, #3024 ) ) ;
#1872=CARTESIAN_POINT ( 'NONE',  ( -5.000232060827701552, 5.589962382322530843, -0.3381422036129833608 ) ) ;
#1879=ADVANCED_FACE ( 'NONE', ( #1701 ), #2962, .F. ) ;
#1881=DIRECTION ( 'NONE',  ( 0.000000000000000000, 0.000000000000000000, 1.000000000000000000 ) ) ;
#1885=CARTESIAN_POINT ( 'NONE',  ( 0.000000000000000000, -72.50000000000001421, -2.500000000000000444 ) ) ;
#1888=CARTESIAN_POINT ( 'NONE',  ( -0.3369232893658926642, -7.494324649304657804, -4.991499248304590353 ) ) ;
#1893=ORIENTED_EDGE ( 'NONE', *, *, #1517, .T. ) ;
#1895=VERTEX_POINT ( 'NONE', #3182 ) ;
#1896=B_SPLINE_CURVE_WITH_KNOTS ( 'NONE', 3,
 ( #537, #2583, #265, #2339, #1545, #2551, #1075, #1592, #1288, #1040, #2606, #2355, #2304, #2053, #3061, #924, #1142, #1359, #2408, #655, #1870, #896, #2373, #2177, #2424, #148, #2640, #1111, #385, #2879, #2625, #1922, #2128, #418, #668, #1425, #640, #1888, #1641, #351 ),
 .UNSPECIFIED., .F., .F.,
 ( 4, 2, 2, 2, 2, 2, 2, 2, 2, 2, 2, 2, 2, 2, 2, 2, 2, 2, 2, 4 ),
 ( 0.000000000000000000, 0.001009991476537153501, 0.002019982953074307436, 0.003029974429611462239, 0.004039965906148617475, 0.005049957382685771844, 0.006059948859222927947, 0.007069940335760082316, 0.007574936074028659934, 0.008079931812297236685, 0.009089923288834390186, 0.01009991476537154195, 0.01110990624190869892, 0.01211989771844585242, 0.01312988919498300593, 0.01363488493325158528, 0.01413988067152016116, 0.01514987214805731987, 0.01565486788632589749, 0.01615986362459447684 ),
 .UNSPECIFIED. ) ;
#1897=CARTESIAN_POINT ( 'NONE',  ( -1.464466094067259139, -67.50000000000000000, 2.499999999999997780 ) ) ;
#1898=EDGE_CURVE ( 'NONE', #1146, #2611, #2608, .T. ) ;
#1900=DIRECTION ( 'NONE',  ( 1.000000000000000000, 0.000000000000000000, -0.000000000000000000 ) ) ;
#1903=DIRECTION ( 'NONE',  ( -0.000000000000000000, -0.000000000000000000, 1.000000000000000000 ) ) ;
#1908=CIRCLE ( 'NONE', #1962, 2.500000000000000444 ) ;
#1911=VERTEX_POINT ( 'NONE', #1223 ) ;
#1912=CARTESIAN_POINT ( 'NONE',  ( -1.997648066307399439, -71.53698439035578360, -4.589990637419044006 ) ) ;
#1915=CARTESIAN_POINT ( 'NONE',  ( -0.1655869666764216153, -67.50000000000001421, -5.000000000000000000 ) ) ;
#1920=CARTESIAN_POINT ( 'NONE',  ( -4.996981400519024952, -48.50997913539912076, 0.1986267936440539450 ) ) ;
#1922=CARTESIAN_POINT ( 'NONE',  ( -2.257837506661119154, -7.153666188643283519, -4.464160652961850495 ) ) ;
#1924=EDGE_CURVE ( 'NONE', #2713, #821, #2239, .T. ) ;
#1926=VERTEX_POINT ( 'NONE', #2911 ) ;
#1928=EDGE_CURVE ( 'NONE', #2713, #97, #773, .T. ) ;
#1930=CARTESIAN_POINT ( 'NONE',  ( 4.965855707945498132, -5.621220898751191797, -0.6727113530297602617 ) ) ;
#1932=CARTESIAN_POINT ( 'NONE',  ( 0.3471650268615566470, -64.00752696620394033, 4.990975288187766701 ) ) ;
#1935=CARTESIAN_POINT ( 'NONE',  ( 2.594030646330690359, -75.41843215906500575, 4.286313293421137871 ) ) ;
#1938=CARTESIAN_POINT ( 'NONE',  ( 4.784761898981735762, -49.60847529508066600, 1.451366868840367808 ) ) ;
#1939=VECTOR ( 'NONE', #1203, 1000.000000000000000 ) ;
#1943=EDGE_LOOP ( 'NONE', ( #1856, #471, #579 ) ) ;
#1945=( LENGTH_UNIT ( ) NAMED_UNIT ( * ) SI_UNIT ( .MILLI., .METRE. ) );
#1949=ORIENTED_EDGE ( 'NONE', *, *, #2025, .T. ) ;
#1950=CARTESIAN_POINT ( 'NONE',  ( 5.000000000000000000, -66.68337520964459486, 0.1770536369485830597 ) ) ;
#1954=CARTESIAN_POINT ( 'NONE',  ( 8.572527594031472993E-15, -70.00000000000000000, 10.00000000000000000 ) ) ;
#1958=DIRECTION ( 'NONE',  ( -0.000000000000000000, -0.000000000000000000, 1.000000000000000000 ) ) ;
#1960=MECHANICAL_DESIGN_GEOMETRIC_PRESENTATION_REPRESENTATION('',(#480),#425);
#1962=AXIS2_PLACEMENT_3D ( 'NONE', #2740, #516, #1214 ) ;
#1965=EDGE_CURVE ( 'NONE', #123, #821, #999, .T. ) ;
#1968=DIRECTION ( 'NONE',  ( 0.000000000000000000, 0.000000000000000000, 1.000000000000000000 ) ) ;
#1970=CARTESIAN_POINT ( 'NONE',  ( -7.500000000000000000, 0.000000000000000000, 10.00000000000000000 ) ) ;
#1971=DIRECTION ( 'NONE',  ( -0.000000000000000000, -0.000000000000000000, -1.000000000000000000 ) ) ;
#1972=DIRECTION ( 'NONE',  ( 0.000000000000000000, 0.000000000000000000, 1.000000000000000000 ) ) ;
#1973=ORIENTED_EDGE ( 'NONE', *, *, #291, .T. ) ;
#1974=CARTESIAN_POINT ( 'NONE',  ( -4.772823865982902092, -49.80222060004894757, -1.490154340647099174 ) ) ;
#1979=VERTEX_POINT ( 'NONE', #2680 ) ;
#1981=CARTESIAN_POINT ( 'NONE',  ( -6.610444160707455418E-15, -72.50000000000009948, -5.000000000000047962 ) ) ;
#1982=FACE_OUTER_BOUND ( 'NONE', #135, .T. ) ;
#1987=CARTESIAN_POINT ( 'NONE',  ( 4.325820249441205689, -74.16453108894374679, 2.526170042365373014 ) ) ;
#1988=ADVANCED_FACE ( 'NONE', ( #3129, #96 ), #2419, .F. ) ;
#1991=LINE ( 'NONE', #1703, #193 ) ;
#1999=DIRECTION ( 'NONE',  ( -0.000000000000000000, -1.000000000000000000, -0.000000000000000000 ) ) ;
#2000=CIRCLE ( 'NONE', #304, 2.500000000000000000 ) ;
#2003=DIRECTION ( 'NONE',  ( 1.000000000000000000, -0.000000000000000000, -0.000000000000000000 ) ) ;
#2004=EDGE_CURVE ( 'NONE', #2753, #810, #669, .T. ) ;
#2008=DIRECTION ( 'NONE',  ( -1.000000000000000000, 0.000000000000000000, 0.000000000000000000 ) ) ;
#2009=ADVANCED_FACE ( 'NONE', ( #1635, #2366 ), #2874, .F. ) ;
#2013=ORIENTED_EDGE ( 'NONE', *, *, #3087, .T. ) ;
#2016=PRODUCT_CONTEXT ( 'NONE', #2986, 'mechanical' ) ;
#2018=CARTESIAN_POINT ( 'NONE',  ( 2.541265623391468331, -7.062137256042765543, 4.317949725309306430 ) ) ;
#2019=CARTESIAN_POINT ( 'NONE',  ( -4.856148773929144902, -50.91572476600896380, 1.192039989181127080 ) ) ;
#2020=DIRECTION ( 'NONE',  ( 0.000000000000000000, 1.000000000000000000, 0.000000000000000000 ) ) ;
#2024=ORIENTED_EDGE ( 'NONE', *, *, #98, .F. ) ;
#2025=EDGE_CURVE ( 'NONE', #1036, #903, #1620, .T. ) ;
#2028=CARTESIAN_POINT ( 'NONE',  ( 4.815309899926791815, -50.66728354398328094, -1.346969744587360074 ) ) ;
#2029=DIRECTION ( 'NONE',  ( 0.000000000000000000, 1.000000000000000000, 0.000000000000000000 ) ) ;
#2030=EDGE_CURVE ( 'NONE', #1911, #1630, #395, .T. ) ;
#2031=CARTESIAN_POINT ( 'NONE',  ( -4.977308113077120844, -51.42299734723061277, 0.4845947803478808380 ) ) ;
#2034=DIRECTION ( 'NONE',  ( 1.000000000000000000, 0.000000000000000000, -0.000000000000000000 ) ) ;
#2037=ORIENTED_EDGE ( 'NONE', *, *, #929, .F. ) ;
#2042=ORIENTED_EDGE ( 'NONE', *, *, #2132, .F. ) ;
#2043=CARTESIAN_POINT ( 'NONE',  ( 4.856137924134493744, -50.91569030856719280, -1.192091538463844191 ) ) ;
#2044=CARTESIAN_POINT ( 'NONE',  ( -0.6937423435388923032, -75.96229638456773614, 4.954702760404292583 ) ) ;
#2050=ORIENTED_EDGE ( 'NONE', *, *, #2030, .T. ) ;
#2051=DIRECTION ( 'NONE',  ( 0.000000000000000000, 0.000000000000000000, 1.000000000000000000 ) ) ;
#2053=CARTESIAN_POINT ( 'NONE',  ( -4.728889495302424528, -5.823500886956166411, 1.655898480698586139 ) ) ;
#2055=DIRECTION ( 'NONE',  ( -0.000000000000000000, -0.000000000000000000, -1.000000000000000000 ) ) ;
#2057=AXIS2_PLACEMENT_3D ( 'NONE', #3145, #2650, #2120 ) ;
#2058=ORIENTED_EDGE ( 'NONE', *, *, #1965, .F. ) ;
#2060=CARTESIAN_POINT ( 'NONE',  ( -4.475554532957456644, -74.00082003167284483, 2.251442214368888362 ) ) ;
#2065=AXIS2_PLACEMENT_3D ( 'NONE', #1383, #1631, #374 ) ;
#2067=CARTESIAN_POINT ( 'NONE',  ( 6.123233995736765296E-16, -80.00000000000000000, -4.999999999999999112 ) ) ;
#2069=ORIENTED_EDGE ( 'NONE', *, *, #1789, .F. ) ;
#2070=CARTESIAN_POINT ( 'NONE',  ( 4.999999999999999112, -73.31662479035541935, 0.000000000000000000 ) ) ;
#2073=CARTESIAN_POINT ( 'NONE',  ( 1.464466094067265800, -72.50000000000001421, -2.499999999999999556 ) ) ;
#2074=ORIENTED_EDGE ( 'NONE', *, *, #942, .T. ) ;
#2075=CARTESIAN_POINT ( 'NONE',  ( 6.124525076959063726E-16, 7.500000000000000000, -4.999999999999999112 ) ) ;
#2079=B_SPLINE_CURVE_WITH_KNOTS ( 'NONE', 3,
 ( #324, #1774, #1513, #1824, #270, #2262, #2831, #3083, #287, #1279, #577, #1580, #3018, #2327, #1808, #2814, #2031, #2524, #3047, #1261, #2019, #24, #3030, #525, #1066, #2592, #3272, #1550 ),
 .UNSPECIFIED., .F., .F.,
 ( 4, 2, 2, 2, 2, 2, 2, 2, 2, 2, 2, 2, 2, 4 ),
 ( 0.000000000000000000, 0.0002948077093299257545, 0.0005896154186598515090, 0.0008844231279897772635, 0.001179230837319703018, 0.001768846255979540866, 0.002358461674639378714, 0.002653269383969297963, 0.002948077093299216345, 0.003537692511959054844, 0.003832500221288973660, 0.004127307930618892041, 0.004422115639948811724, 0.004716923349278730540 ),
 .UNSPECIFIED. ) ;
#2080=CARTESIAN_POINT ( 'NONE',  ( -2.309991845038993574, -75.54707137493313951, 4.447043502685488647 ) ) ;
#2083=VERTEX_POINT ( 'NONE', #2202 ) ;
#2087=EDGE_CURVE ( 'NONE', #1541, #1748, #1364, .T. ) ;
#2089=DIRECTION ( 'NONE',  ( 0.000000000000000000, 0.000000000000000000, 1.000000000000000000 ) ) ;
#2091=DIRECTION ( 'NONE',  ( -0.000000000000000000, -0.000000000000000000, -1.000000000000000000 ) ) ;
#2092=ORIENTED_EDGE ( 'NONE', *, *, #1758, .F. ) ;
#2093=FACE_OUTER_BOUND ( 'NONE', #2388, .T. ) ;
#2098=ORIENTED_EDGE ( 'NONE', *, *, #320, .F. ) ;
#2099=CARTESIAN_POINT ( 'NONE',  ( 2.500000000000004441, -70.00000000000000000, 0.000000000000000000 ) ) ;
#2101=VERTEX_POINT ( 'NONE', #2463 ) ;
#2102=AXIS2_PLACEMENT_3D ( 'NONE', #1954, #479, #2203 ) ;
#2103=DIRECTION ( 'NONE',  ( 0.000000000000000000, 0.000000000000000000, 1.000000000000000000 ) ) ;
#2104=DIRECTION ( 'NONE',  ( 1.000000000000000000, 0.000000000000000000, 0.000000000000000000 ) ) ;
#2106=CARTESIAN_POINT ( 'NONE',  ( 4.480628327518417109, 6.016609984030584890, -2.242680489316260850 ) ) ;
#2107=CARTESIAN_POINT ( 'NONE',  ( -0.1739454948912136090, -64.00000000000001421, 5.000000000000000000 ) ) ;
#2109=VERTEX_POINT ( 'NONE', #2499 ) ;
#2110=CARTESIAN_POINT ( 'NONE',  ( -0.8431454290909620175, 7.454306392314355989, -4.931260737871609123 ) ) ;
#2113=CARTESIAN_POINT ( 'NONE',  ( -4.990448535730164004, -73.33113742485521414, 0.3539254956240150962 ) ) ;
#2115=DIRECTION ( 'NONE',  ( 0.000000000000000000, 0.000000000000000000, 1.000000000000000000 ) ) ;
#2116=ORIENTED_EDGE ( 'NONE', *, *, #986, .F. ) ;
#2118=CARTESIAN_POINT ( 'NONE',  ( -2.499999999999992006, -69.83441493831065827, -4.330127018922196314 ) ) ;
#2120=DIRECTION ( 'NONE',  ( 1.000000000000000000, 0.000000000000000000, 0.000000000000000000 ) ) ;
#2121=COLOUR_RGB ( '',0.8941176470588234615, 0.8941176470588234615, 0.8941176470588234615 ) ;
#2122=EDGE_LOOP ( 'NONE', ( #1421, #1079, #2069, #1710 ) ) ;
#2123=CARTESIAN_POINT ( 'NONE',  ( -2.499999999999995559, -71.46446609406727646, -1.464466094067262025 ) ) ;
#2126=CARTESIAN_POINT ( 'NONE',  ( 4.733269301232542858, 5.819947390767942430, -1.643717648664120068 ) ) ;
#2127=CARTESIAN_POINT ( 'NONE',  ( -5.000000000000000888, -66.68337520964462328, 0.3546751931833541649 ) ) ;
#2128=CARTESIAN_POINT ( 'NONE',  ( -2.108823893667861604, -7.199131270151879924, -4.536514892156152889 ) ) ;
#2129=ORIENTED_EDGE ( 'NONE', *, *, #3177, .T. ) ;
#2130=CARTESIAN_POINT ( 'NONE',  ( -2.499999999999999556, 0.000000000000000000, 10.00000000000000000 ) ) ;
#2132=EDGE_CURVE ( 'NONE', #651, #1093, #1372, .T. ) ;
#2134=PRODUCT_DEFINITION_SHAPE ( 'NONE', 'NONE',  #1648 ) ;
#2135=CARTESIAN_POINT ( 'NONE',  ( -1.658049672226218574, -71.87792464909678358, -4.718635845934137762 ) ) ;
#2138=CARTESIAN_POINT ( 'NONE',  ( 8.572527594031472993E-15, -70.00000000000000000, 10.00000000000000000 ) ) ;
#2141=CARTESIAN_POINT ( 'NONE',  ( -1.464466094067257806, -72.50000000000001421, -2.499999999999999556 ) ) ;
#2144=CARTESIAN_POINT ( 'NONE',  ( -0.6741883319902871596, 7.471549563736964217, -4.957238835368188212 ) ) ;
#2147=EDGE_CURVE ( 'NONE', #216, #1541, #2250, .T. ) ;
#2148=CARTESIAN_POINT ( 'NONE',  ( -2.500000000000000000, 0.000000000000000000, -10.00000000000000000 ) ) ;
#2151=CARTESIAN_POINT ( 'NONE',  ( -2.499999999999994671, -68.53553390593273775, 1.464466094067261137 ) ) ;
#2154=ORIENTED_EDGE ( 'NONE', *, *, #1758, .T. ) ;
#2155=VECTOR ( 'NONE', #412, 1000.000000000000000 ) ;
#2159=PRODUCT ( 'Needle Bar', 'Needle Bar', '', ( #2016 ) ) ;
#2160=CARTESIAN_POINT ( 'NONE',  ( -4.324630367402185982, 6.131366064188266130, 2.529815037953009327 ) ) ;
#2166=VERTEX_POINT ( 'NONE', #714 ) ;
#2167=CARTESIAN_POINT ( 'NONE',  ( -1.653533745081442907, -68.11807823234784109, -4.720230888861525642 ) ) ;
#2168=AXIS2_PLACEMENT_3D ( 'NONE', #1249, #2020, #1972 ) ;
#2170=DIRECTION ( 'NONE',  ( -0.000000000000000000, -1.000000000000000000, -0.000000000000000000 ) ) ;
#2175=AXIS2_PLACEMENT_3D ( 'NONE', #505, #819, #2543 ) ;
#2177=CARTESIAN_POINT ( 'NONE',  ( -4.480628327518417109, -6.016609984030584890, -2.242680489316260850 ) ) ;
#2183=CARTESIAN_POINT ( 'NONE',  ( 0.1666858246784454212, -72.50000000000002842, -5.000000000000003553 ) ) ;
#2184=CARTESIAN_POINT ( 'NONE',  ( 4.725421832813011314, -5.824466512821798503, -1.642406358834817004 ) ) ;
#2186=CARTESIAN_POINT ( 'NONE',  ( 8.572527594031472993E-15, -70.00000000000000000, 10.00000000000000000 ) ) ;
#2188=CARTESIAN_POINT ( 'NONE',  ( 0.1654076819047616553, -67.50000000000000000, -4.999999999999998224 ) ) ;
#2190=CARTESIAN_POINT ( 'NONE',  ( -4.945771905224659371, -48.69008891295303698, -0.7565992915569080823 ) ) ;
#2200=CARTESIAN_POINT ( 'NONE',  ( 4.990448535730164004, -66.66886257514475744, 0.3539254956240222016 ) ) ;
#2202=CARTESIAN_POINT ( 'NONE',  ( -2.499999999999991118, -70.00000000000000000, -4.330127018922196314 ) ) ;
#2203=DIRECTION ( 'NONE',  ( 1.000000000000000000, 0.000000000000000000, -0.000000000000000000 ) ) ;
#2204=CARTESIAN_POINT ( 'NONE',  ( -4.999998311775604165, -48.50000562741465870, 0.09894250604207632804 ) ) ;
#2206=CARTESIAN_POINT ( 'NONE',  ( 4.945777185212984151, -48.69007577354707905, -0.7564652374250301348 ) ) ;
#2207=AXIS2_PLACEMENT_3D ( 'NONE', #2921, #394, #3191 ) ;
#2218=CARTESIAN_POINT ( 'NONE',  ( 1.373679055183318676, -64.14932959975399740, 4.819953665648758268 ) ) ;
#2220=CARTESIAN_POINT ( 'NONE',  ( 0.000000000000000000, -67.50000000000000000, -2.500000000000000444 ) ) ;
#2222=CARTESIAN_POINT ( 'NONE',  ( -4.856137924134493744, -49.08430969143282141, -1.192091538463844191 ) ) ;
#2224=CARTESIAN_POINT ( 'NONE',  ( 4.793520869840776299, -49.51425668076524289, -1.422568331971221456 ) ) ;
#2225=CARTESIAN_POINT ( 'NONE',  ( 0.000000000000000000, -80.00000000000000000, 0.000000000000000000 ) ) ;
#2229=ORIENTED_EDGE ( 'NONE', *, *, #1924, .T. ) ;
#2231=CARTESIAN_POINT ( 'NONE',  ( 2.483169110057957596, -70.33326608521694823, -4.339962428766264146 ) ) ;
#2232=CARTESIAN_POINT ( 'NONE',  ( 3.772047191027663615, -6.487346954507292374, -3.297239103104800506 ) ) ;
#2238=CARTESIAN_POINT ( 'NONE',  ( 4.724063086364460595, -73.70412200079239540, 1.668329630282858078 ) ) ;
#2239=LINE ( 'NONE', #3245, #2902 ) ;
#2244=ORIENTED_EDGE ( 'NONE', *, *, #3154, .F. ) ;
#2246=CARTESIAN_POINT ( 'NONE',  ( 4.669423702320314895, -5.869651582198522455, -1.795146503317839759 ) ) ;
#2250=LINE ( 'NONE', #2716, #3222 ) ;
#2252=DIRECTION ( 'NONE',  ( 0.000000000000000000, 1.000000000000000000, 0.000000000000000000 ) ) ;
#2256=VECTOR ( 'NONE', #2348, 1000.000000000000000 ) ;
#2258=VERTEX_POINT ( 'NONE', #254 ) ;
#2262=CARTESIAN_POINT ( 'NONE',  ( -4.815279722017292485, -50.66710047508086490, -1.347079874192880444 ) ) ;
#2265=CARTESIAN_POINT ( 'NONE',  ( 6.124525076959063726E-16, 7.500000000000000000, -4.999999999999999112 ) ) ;
#2268=CARTESIAN_POINT ( 'NONE',  ( 4.985642101603771081, -48.54846037558075267, 0.3907762206522687465 ) ) ;
#2274=AXIS2_PLACEMENT_3D ( 'NONE', #155, #932, #916 ) ;
#2275=CARTESIAN_POINT ( 'NONE',  ( 2.108823893667861604, 7.199131270151879924, -4.536514892156152889 ) ) ;
#2277=CIRCLE ( 'NONE', #1743, 2.500000000000000444 ) ;
#2281=CARTESIAN_POINT ( 'NONE',  ( -2.499999999999999556, 0.000000000000000000, -10.00000000000000000 ) ) ;
#2283=CARTESIAN_POINT ( 'NONE',  ( 0.000000000000000000, 0.000000000000000000, 10.00000000000000000 ) ) ;
#2287=ORIENTED_EDGE ( 'NONE', *, *, #2030, .F. ) ;
#2293=CARTESIAN_POINT ( 'NONE',  ( 4.784702204231576772, -50.39069709306253486, -1.451562066005745999 ) ) ;
#2294=CARTESIAN_POINT ( 'NONE',  ( -4.999999999999999112, -66.68337520964460907, 0.000000000000000000 ) ) ;
#2295=CARTESIAN_POINT ( 'NONE',  ( 0.000000000000000000, 80.00000000000000000, 4.999999999999999112 ) ) ;
#2296=UNCERTAINTY_MEASURE_WITH_UNIT (LENGTH_MEASURE( 1.000000000000000082E-05 ), #2905, 'distance_accuracy_value', 'NONE');
#2298=CARTESIAN_POINT ( 'NONE',  ( 3.061616997868383634E-16, -60.00000000000000000, 2.500000000000000444 ) ) ;
#2300=DIRECTION ( 'NONE',  ( 0.000000000000000000, -1.000000000000000000, 0.000000000000000000 ) ) ;
#2302=ORIENTED_EDGE ( 'NONE', *, *, #1778, .T. ) ;
#2304=CARTESIAN_POINT ( 'NONE',  ( -4.476439251420855747, -6.019721759973592157, 2.250752599798611975 ) ) ;
#2305=ORIENTED_EDGE ( 'NONE', *, *, #553, .T. ) ;
#2306=CARTESIAN_POINT ( 'NONE',  ( 2.499999999999999556, 3.061616997868382648E-16, -10.00000000000000000 ) ) ;
#2309=AXIS2_PLACEMENT_3D ( 'NONE', #535, #782, #2550 ) ;
#2311=CARTESIAN_POINT ( 'NONE',  ( -3.790413940515794611, -74.65884673497926372, 3.275345238443577500 ) ) ;
#2312=B_SPLINE_CURVE_WITH_KNOTS ( 'NONE', 3,
 ( #1168, #1463, #2694, #1709, #2725, #3252, #456, #2496, #2741, #218, #426, #2232, #2675, #3238, #1231, #2246, #2184, #979, #406, #1930, #2542, #524, #65, #1074, #82, #1091, #251, #851, #1528, #1834, #1510, #1259, #3017, #2018, #831, #2779, #756, #2522, #1745, #1499 ),
 .UNSPECIFIED., .F., .F.,
 ( 4, 2, 2, 2, 2, 2, 2, 2, 2, 2, 2, 2, 2, 2, 2, 2, 2, 2, 2, 4 ),
 ( 0.01615986362459447684, 0.01666419217584455895, 0.01716852072709463758, 0.01817717782959479833, 0.01918583493209496255, 0.02019449203459512329, 0.02120314913709528404, 0.02221180623959544478, 0.02271613479084552342, 0.02322046334209560553, 0.02422912044459576628, 0.02523777754709592702, 0.02574210609834600566, 0.02624643464959608777, 0.02725509175209624851, 0.02826374885459641273, 0.02927240595709657001, 0.03028106305959672728, 0.03128972016209689150, 0.03229837726459704877 ),
 .UNSPECIFIED. ) ;
#2313=CARTESIAN_POINT ( 'NONE',  ( 8.572527594031472993E-15, -70.00000000000000000, 0.000000000000000000 ) ) ;
#2316=CYLINDRICAL_SURFACE ( 'NONE', #1246, 1.500000000000000444 ) ;
#2320=CARTESIAN_POINT ( 'NONE',  ( 6.000000000000010658, -70.00000000000000000, 10.00000000000000000 ) ) ;
#2326=EDGE_LOOP ( 'NONE', ( #1723, #628 ) ) ;
#2327=CARTESIAN_POINT ( 'NONE',  ( -5.000012828558699773, -51.50004276186603391, 0.09784062508662537405 ) ) ;
#2328=CIRCLE ( 'NONE', #1053, 7.500000000000000000 ) ;
#2336=DIRECTION ( 'NONE',  ( 0.000000000000000000, 0.000000000000000000, 1.000000000000000000 ) ) ;
#2339=CARTESIAN_POINT ( 'NONE',  ( -1.331840593602624745, -7.388197954259797307, 4.830944097608436572 ) ) ;
#2340=ORIENTED_EDGE ( 'NONE', *, *, #2617, .F. ) ;
#2341=CARTESIAN_POINT ( 'NONE',  ( -3.320170879781855433, 6.729821324027721374, 3.751849819826997834 ) ) ;
#2348=DIRECTION ( 'NONE',  ( -0.000000000000000000, -1.000000000000000000, -0.000000000000000000 ) ) ;
#2351=DIRECTION ( 'NONE',  ( 0.000000000000000000, -1.000000000000000000, 0.000000000000000000 ) ) ;
#2353=CARTESIAN_POINT ( 'NONE',  ( 1.654849718955805127, 7.321828482412975347, 4.729586325473386310 ) ) ;
#2355=CARTESIAN_POINT ( 'NONE',  ( -4.324727228821070746, -6.131211258369285488, 2.529220782163199122 ) ) ;
#2357=CARTESIAN_POINT ( 'NONE',  ( -2.259265036967212481, 7.158401641891561695, 4.472413388026437175 ) ) ;
#2359=ORIENTED_EDGE ( 'NONE', *, *, #3194, .F. ) ;
#2360=CARTESIAN_POINT ( 'NONE',  ( -0.6584138513982479290, -72.41738593900605281, -4.959126935340800735 ) ) ;
#2364=FACE_OUTER_BOUND ( 'NONE', #1871, .T. ) ;
#2365=ADVANCED_FACE ( 'NONE', ( #288 ), #1762, .F. ) ;
#2366=FACE_BOUND ( 'NONE', #658, .T. ) ;
#2371=DIRECTION ( 'NONE',  ( -0.000000000000000000, -1.000000000000000000, -0.000000000000000000 ) ) ;
#2372=DIRECTION ( 'NONE',  ( 0.000000000000000000, 0.000000000000000000, 1.000000000000000000 ) ) ;
#2373=CARTESIAN_POINT ( 'NONE',  ( -4.733269301232542858, -5.819947390767942430, -1.643717648664120068 ) ) ;
#2375=CARTESIAN_POINT ( 'NONE',  ( -3.971811635560102527, 6.365546751009641291, -3.053863045737025494 ) ) ;
#2376=ADVANCED_FACE ( 'NONE', ( #1982 ), #1216, .F. ) ;
#2384=DIRECTION ( 'NONE',  ( -0.000000000000000000, -0.000000000000000000, 1.000000000000000000 ) ) ;
#2385=( BOUNDED_CURVE ( )  B_SPLINE_CURVE ( 3, ( #363, #2598, #1085, #2099 ),
 .UNSPECIFIED., .F., .T. ) 
 B_SPLINE_CURVE_WITH_KNOTS ( ( 4, 4 ),
 ( 0.000000000000000000, 1.570796326794896780 ),
 .UNSPECIFIED. ) 
 CURVE ( )  GEOMETRIC_REPRESENTATION_ITEM ( )  RATIONAL_B_SPLINE_CURVE ( ( 1.000000000000000000, 0.8047378541243649375, 0.8047378541243649375, 1.000000000000000000 ) ) 
 REPRESENTATION_ITEM ( '' )  );
#2387=CARTESIAN_POINT ( 'NONE',  ( 2.368690460745422222, -69.18407089167581603, -4.403897978979204986 ) ) ;
#2388=EDGE_LOOP ( 'NONE', ( #550, #172, #3082, #1459, #1353 ) ) ;
#2389=DIRECTION ( 'NONE',  ( 0.000000000000000000, 1.000000000000000000, 0.000000000000000000 ) ) ;
#2392=CARTESIAN_POINT ( 'NONE',  ( 0.3421168542193412376, 7.499999999999999112, 4.999999999999999112 ) ) ;
#2395=CARTESIAN_POINT ( 'NONE',  ( -2.541265623391468331, 7.062137256042765543, 4.317949725309306430 ) ) ;
#2397=ORIENTED_EDGE ( 'NONE', *, *, #1289, .F. ) ;
#2399=CARTESIAN_POINT ( 'NONE',  ( -6.610444160707455418E-15, -72.50000000000009948, -5.000000000000047962 ) ) ;
#2400=VERTEX_POINT ( 'NONE', #171 ) ;
#2403=CARTESIAN_POINT ( 'NONE',  ( 0.6585099098572929632, -67.58258473628077923, -4.959140660327080674 ) ) ;
#2405=FACE_OUTER_BOUND ( 'NONE', #1576, .T. ) ;
#2408=CARTESIAN_POINT ( 'NONE',  ( -4.999850703040199740, -5.590303478919644853, 0.1739517833579089512 ) ) ;
#2414=EDGE_CURVE ( 'NONE', #1054, #903, #2328, .T. ) ;
#2415=ORIENTED_EDGE ( 'NONE', *, *, #1285, .F. ) ;
#2416=CARTESIAN_POINT ( 'NONE',  ( -2.241708953382383296, -68.88112708827009101, -4.469887766052389466 ) ) ;
#2417=EDGE_CURVE ( 'NONE', #2549, #2400, #644, .T. ) ;
#2419=PLANE ( 'NONE',  #1159 ) ;
#2421=CARTESIAN_POINT ( 'NONE',  ( 3.061616997868384127E-16, -72.50000000000001421, 2.500000000000000444 ) ) ;
#2422=CLOSED_SHELL ( 'NONE', ( #710, #72, #2697, #2376, #1134, #1821, #2531, #1573, #1512, #2886, #2465, #2009, #2692, #1988, #213, #165, #609, #1130, #1879, #1715, #54, #105, #2365, #1739, #1373, #2892, #757, #22 ) ) ;
#2424=CARTESIAN_POINT ( 'NONE',  ( -4.325873777034227707, -6.130418473463322471, -2.527359400829327196 ) ) ;
#2429=DIRECTION ( 'NONE',  ( -0.000000000000000000, -0.000000000000000000, -1.000000000000000000 ) ) ;
#2430=EDGE_LOOP ( 'NONE', ( #2397, #2415, #1766, #1597 ) ) ;
#2434=DIRECTION ( 'NONE',  ( 0.000000000000000000, 0.000000000000000000, -1.000000000000000000 ) ) ;
#2435=AXIS2_PLACEMENT_3D ( 'NONE', #1432, #3188, #2459 ) ;
#2436=CARTESIAN_POINT ( 'NONE',  ( -4.977300154039397739, -48.57702733233907821, 0.4847224211361968460 ) ) ;
#2447=CARTESIAN_POINT ( 'NONE',  ( 0.000000000000000000, -80.00000000000000000, 4.999999999999999112 ) ) ;
#2448=EDGE_CURVE ( 'NONE', #903, #1054, #1108, .T. ) ;
#2451=CARTESIAN_POINT ( 'NONE',  ( 1.375028959113674842, -75.85031115372576949, 4.819517586941451270 ) ) ;
#2452=CARTESIAN_POINT ( 'NONE',  ( -4.945480083184111919, -48.69114140900990151, 0.7590239407556941265 ) ) ;
#2454=CARTESIAN_POINT ( 'NONE',  ( 4.769696007084725409, -49.90026769176149202, -1.500000000000006661 ) ) ;
#2457=ORIENTED_EDGE ( 'NONE', *, *, #482, .T. ) ;
#2459=DIRECTION ( 'NONE',  ( 1.000000000000000000, 0.000000000000000000, 0.000000000000000000 ) ) ;
#2461=CARTESIAN_POINT ( 'NONE',  ( 2.309991845038998903, -64.45292862506686049, 4.447043502685485983 ) ) ;
#2463=CARTESIAN_POINT ( 'NONE',  ( 4.769696007084725409, -50.00000000000000000, -1.500000000000006439 ) ) ;
#2465=ADVANCED_FACE ( 'NONE', ( #2971 ), #1661, .F. ) ;
#2466=CARTESIAN_POINT ( 'NONE',  ( -4.769696007084727185, -49.80352985508882568, 1.499999999999993339 ) ) ;
#2467=( BOUNDED_CURVE ( )  B_SPLINE_CURVE ( 3, ( #623, #2896, #2686, #1177 ),
 .UNSPECIFIED., .F., .F. ) 
 B_SPLINE_CURVE_WITH_KNOTS ( ( 4, 4 ),
 ( 1.570796326794896558, 3.141592653589794448 ),
 .UNSPECIFIED. ) 
 CURVE ( )  GEOMETRIC_REPRESENTATION_ITEM ( )  RATIONAL_B_SPLINE_CURVE ( ( 1.000000000000000000, 0.8047378541243646044, 0.8047378541243646044, 1.000000000000000000 ) ) 
 REPRESENTATION_ITEM ( '' )  );
#2469=CARTESIAN_POINT ( 'NONE',  ( 4.815110478384604598, -49.33416175143172921, 1.347678760471933135 ) ) ;
#2475=ORIENTED_EDGE ( 'NONE', *, *, #2848, .F. ) ;
#2481=DIRECTION ( 'NONE',  ( 0.000000000000000000, 1.000000000000000000, 0.000000000000000000 ) ) ;
#2483=CARTESIAN_POINT ( 'NONE',  ( 2.500000000000004441, -70.00000000000000000, 0.000000000000000000 ) ) ;
#2494=EDGE_LOOP ( 'NONE', ( #1448, #1012 ) ) ;
#2496=CARTESIAN_POINT ( 'NONE',  ( 2.262527220957939456, -7.157552900320828471, -4.471083064257649120 ) ) ;
#2499=CARTESIAN_POINT ( 'NONE',  ( 6.123233995736765296E-16, 80.00000000000000000, -4.999999999999999112 ) ) ;
#2500=CARTESIAN_POINT ( 'NONE',  ( 3.359434976081794311, -74.97862781767101126, 3.716172273690823147 ) ) ;
#2503=CARTESIAN_POINT ( 'NONE',  ( 4.916145513835878944, -48.80134495313303944, 0.9228047480949569392 ) ) ;
#2505=ORIENTED_EDGE ( 'NONE', *, *, #925, .T. ) ;
#2509=CARTESIAN_POINT ( 'NONE',  ( 4.661216347248879899, -66.22080041675921791, 1.816027882404178229 ) ) ;
#2510=EDGE_CURVE ( 'NONE', #1195, #1139, #2312, .T. ) ;
#2517=CARTESIAN_POINT ( 'NONE',  ( 4.945591935980590215, -48.69073257577973379, 0.7581774313040230417 ) ) ;
#2520=VERTEX_POINT ( 'NONE', #350 ) ;
#2522=CARTESIAN_POINT ( 'NONE',  ( 0.6778607859896496057, -7.476644527972223564, 4.965157125901431101 ) ) ;
#2523=CIRCLE ( 'NONE', #1095, 2.499999999999999556 ) ;
#2524=CARTESIAN_POINT ( 'NONE',  ( -4.945591935980590215, -51.30926742422028752, 0.7581774313040230417 ) ) ;
#2527=DIRECTION ( 'NONE',  ( 0.000000000000000000, 0.000000000000000000, 1.000000000000000000 ) ) ;
#2528=DIRECTION ( 'NONE',  ( 1.000000000000000000, 0.000000000000000000, 0.000000000000000000 ) ) ;
#2531=ADVANCED_FACE ( 'NONE', ( #503 ), #6, .T. ) ;
#2533=CARTESIAN_POINT ( 'NONE',  ( 2.500000000000008438, -70.16838717509892831, -4.330127018922188320 ) ) ;
#2535=CYLINDRICAL_SURFACE ( 'NONE', #3156, 4.999999999999999112 ) ;
#2539=AXIS2_PLACEMENT_3D ( 'NONE', #2769, #2429, #965 ) ;
#2541=MECHANICAL_DESIGN_GEOMETRIC_PRESENTATION_REPRESENTATION('',(#590),#375);
#2542=CARTESIAN_POINT ( 'NONE',  ( 5.000232060827701552, -5.589962382322530843, -0.3381422036129833608 ) ) ;
#2543=DIRECTION ( 'NONE',  ( 0.000000000000000000, -0.000000000000000000, -1.000000000000000000 ) ) ;
#2545=LINE ( 'NONE', #41, #1516 ) ;
#2549=VERTEX_POINT ( 'NONE', #2294 ) ;
#2550=DIRECTION ( 'NONE',  ( -1.000000000000000000, 0.000000000000000000, 0.000000000000000000 ) ) ;
#2551=CARTESIAN_POINT ( 'NONE',  ( -2.258341722794894313, -7.158742388247099520, 4.472964013438597952 ) ) ;
#2552=ORIENTED_EDGE ( 'NONE', *, *, #2852, .F. ) ;
#2558=FACE_OUTER_BOUND ( 'NONE', #2816, .T. ) ;
#2561=ORIENTED_EDGE ( 'NONE', *, *, #1289, .T. ) ;
#2562=EDGE_CURVE ( 'NONE', #2549, #3219, #2587, .T. ) ;
#2565=ORIENTED_EDGE ( 'NONE', *, *, #995, .F. ) ;
#2566=CARTESIAN_POINT ( 'NONE',  ( 4.856197996442241482, -50.91599292333928872, 1.191843005749488871 ) ) ;
#2568=B_SPLINE_CURVE_WITH_KNOTS ( 'NONE', 3,
 ( #208, #494, #1222, #160, #2238, #971, #1987, #1173, #2991, #2500, #921, #1935, #2940, #432, #2451, #2717, #177, #1188, #448, #805 ),
 .UNSPECIFIED., .F., .F.,
 ( 4, 2, 2, 2, 2, 2, 2, 2, 2, 4 ),
 ( 0.000000000000000000, 0.001046161093956322419, 0.002092322187912644838, 0.003138483281868968341, 0.004184644375825291411, 0.005230805469781614481, 0.006276966563737938418, 0.007323127657694261487, 0.007846208204672419986, 0.008369288751650577618 ),
 .UNSPECIFIED. ) ;
#2571=CARTESIAN_POINT ( 'NONE',  ( -4.815265823182749649, -73.58047044739645060, 1.356348383020188786 ) ) ;
#2572=AXIS2_PLACEMENT_3D ( 'NONE', #1563, #1281, #2770 ) ;
#2573=DIRECTION ( 'NONE',  ( 1.000000000000000000, 0.000000000000000000, -0.000000000000000000 ) ) ;
#2575=VECTOR ( 'NONE', #1069, 1000.000000000000000 ) ;
#2579=ORIENTED_EDGE ( 'NONE', *, *, #2912, .T. ) ;
#2580=CARTESIAN_POINT ( 'NONE',  ( 0.000000000000000000, -60.00000000000000000, 0.000000000000000000 ) ) ;
#2581=SHAPE_REPRESENTATION_RELATIONSHIP ( 'NONE' , 'NONE' ,  #457, #3218 ) ;
#2583=CARTESIAN_POINT ( 'NONE',  ( -0.3421168542193412376, -7.499999999999999112, 4.999999999999999112 ) ) ;
#2587=B_SPLINE_CURVE_WITH_KNOTS ( 'NONE', 3,
 ( #1014, #2127, #1358, #3029, #1772, #233, #269, #490, #1278, #3095, #1245, #587, #1591, #998, #333, #2863, #2605, #101, #2107, #1339 ),
 .UNSPECIFIED., .F., .F.,
 ( 4, 2, 2, 2, 2, 2, 2, 2, 2, 4 ),
 ( 0.000000000000000000, 0.001046161093956322419, 0.002092322187912644404, 0.003138483281868967040, 0.004184644375825288809, 0.005230805469781612746, 0.006276966563737934948, 0.007323127657694257150, 0.007846208204672414782, 0.008369288751650572414 ),
 .UNSPECIFIED. ) ;
#2588=EDGE_CURVE ( 'NONE', #1748, #123, #3114, .T. ) ;
#2591=ORIENTED_EDGE ( 'NONE', *, *, #1898, .T. ) ;
#2592=CARTESIAN_POINT ( 'NONE',  ( -4.772817378855775949, -50.19781530912092649, 1.490176662683681652 ) ) ;
#2596=VECTOR ( 'NONE', #1182, 1000.000000000000000 ) ;
#2598=CARTESIAN_POINT ( 'NONE',  ( 1.464466094067265800, -72.50000000000001421, 2.499999999999999556 ) ) ;
#2600=EDGE_LOOP ( 'NONE', ( #1693, #3235, #1600, #2287, #665 ) ) ;
#2602=DIRECTION ( 'NONE',  ( 0.000000000000000000, 1.000000000000000000, 0.000000000000000000 ) ) ;
#2604=CARTESIAN_POINT ( 'NONE',  ( 4.829496642845706234, 5.738802261244866365, 1.336683695250854953 ) ) ;
#2605=CARTESIAN_POINT ( 'NONE',  ( -0.6967678811844660869, -64.03802537814742379, 4.954315763534758332 ) ) ;
#2606=CARTESIAN_POINT ( 'NONE',  ( -3.971188403759415397, -6.365899760466498414, 3.054486213830300390 ) ) ;
#2608=B_SPLINE_CURVE_WITH_KNOTS ( 'NONE', 3,
 ( #1667, #2466, #701, #1190, #938, #2718, #416, #2924, #2452, #2436, #465, #1920, #2204, #666, #162, #1174, #192, #2190, #2941, #684, #2222, #434, #1439, #3229, #957, #1974, #449, #178 ),
 .UNSPECIFIED., .F., .F.,
 ( 4, 2, 2, 2, 2, 2, 2, 2, 2, 2, 2, 2, 2, 4 ),
 ( 0.004716923349278730540, 0.005306377133062306975, 0.005601104024954096060, 0.005895830916845884277, 0.006485284700629445967, 0.006780011592521222909, 0.007074738484412999850, 0.007369465376304777660, 0.007664192268196553734, 0.008253646051980109352, 0.008548372943871894100, 0.008843099835763678848, 0.009137826727655463596, 0.009432553619547248344 ),
 .UNSPECIFIED. ) ;
#2609=CARTESIAN_POINT ( 'NONE',  ( -4.722607672194940598, 5.826754641390677669, 1.650547109183062355 ) ) ;
#2611=VERTEX_POINT ( 'NONE', #604 ) ;
#2616=CARTESIAN_POINT ( 'NONE',  ( -0.6589706823815268955, -67.58264602806174537, -4.959110006177418484 ) ) ;
#2617=EDGE_CURVE ( 'NONE', #2083, #2753, #1518, .T. ) ;
#2618=LINE ( 'NONE', #1334, #2575 ) ;
#2621=DIRECTION ( 'NONE',  ( 0.000000000000000000, 0.000000000000000000, -1.000000000000000000 ) ) ;
#2623=CARTESIAN_POINT ( 'NONE',  ( 3.061616997868383634E-16, -60.00000000000000000, 2.500000000000000444 ) ) ;
#2625=CARTESIAN_POINT ( 'NONE',  ( -2.543753134549881167, -7.057059595574596500, -4.307653715470421751 ) ) ;
#2626=EDGE_LOOP ( 'NONE', ( #1478, #1041, #2726, #2050, #2690 ) ) ;
#2629=CARTESIAN_POINT ( 'NONE',  ( -1.120846245543385855, -72.24071170040616607, -4.875204307872176734 ) ) ;
#2630=CARTESIAN_POINT ( 'NONE',  ( 0.000000000000000000, 0.000000000000000000, 10.00000000000000000 ) ) ;
#2631=EDGE_LOOP ( 'NONE', ( #346, #2042 ) ) ;
#2633=B_SPLINE_CURVE_WITH_KNOTS ( 'NONE', 3,
 ( #2399, #2644, #840, #2360, #3155, #2629, #1840, #1598, #2135, #1912, #902, #646, #2918, #89, #1647, #358 ),
 .UNSPECIFIED., .F., .F.,
 ( 4, 2, 2, 2, 2, 2, 2, 4 ),
 ( 0.003977372743944438890, 0.004474137685135931054, 0.004970902626327423218, 0.005467667567518916250, 0.005964432508710407546, 0.006957962391093391874, 0.007454727332284884038, 0.007951492273476376202 ),
 .UNSPECIFIED. ) ;
#2638=CARTESIAN_POINT ( 'NONE',  ( 1.331840593602624745, 7.388197954259797307, 4.830944097608436572 ) ) ;
#2640=CARTESIAN_POINT ( 'NONE',  ( -3.769434200324356166, -6.488926209160664094, -3.300387065219955840 ) ) ;
#2641=CARTESIAN_POINT ( 'NONE',  ( -3.326284669807233918, 6.726800191391157924, -3.746459129603366467 ) ) ;
#2644=CARTESIAN_POINT ( 'NONE',  ( -0.1665494872612699462, -72.50000000000004263, -5.000000000000003553 ) ) ;
#2645=CIRCLE ( 'NONE', #205, 4.999999999999999112 ) ;
#2646=EDGE_LOOP ( 'NONE', ( #2098, #2591, #3244, #2305 ) ) ;
#2648=CARTESIAN_POINT ( 'NONE',  ( -1.880783153433909227, -68.34517127307829298, -4.634372473166646245 ) ) ;
#2649=CARTESIAN_POINT ( 'NONE',  ( 7.500000000000000000, 9.184850993605147944E-16, -10.00000000000000000 ) ) ;
#2650=DIRECTION ( 'NONE',  ( -0.000000000000000000, -0.000000000000000000, 1.000000000000000000 ) ) ;
#2656=CARTESIAN_POINT ( 'NONE',  ( -1.334319281011194347, 7.387780498848168342, 4.830307711356911504 ) ) ;
#2663=DIRECTION ( 'NONE',  ( 0.000000000000000000, 1.000000000000000000, 0.000000000000000000 ) ) ;
#2665=CARTESIAN_POINT ( 'NONE',  ( -2.499999999999995559, -71.46446609406727646, 1.464466094067262025 ) ) ;
#2667=EDGE_CURVE ( 'NONE', #2258, #2713, #219, .T. ) ;
#2670=MANIFOLD_SOLID_BREP ( 'Cut-Extrude2', #2422 ) ;
#2671=CARTESIAN_POINT ( 'NONE',  ( -2.547727811071581527, 7.059815111224851947, -4.314169979798982091 ) ) ;
#2675=CARTESIAN_POINT ( 'NONE',  ( 3.971811635560102527, -6.365546751009641291, -3.053863045737025494 ) ) ;
#2677=CARTESIAN_POINT ( 'NONE',  ( -2.164506549894624321, -68.73869660040230656, -4.508290309894544379 ) ) ;
#2680=CARTESIAN_POINT ( 'NONE',  ( 3.061616997868383634E-16, -80.00000000000000000, 2.500000000000000444 ) ) ;
#2682=AXIS2_PLACEMENT_3D ( 'NONE', #486, #2336, #1072 ) ;
#2683=CARTESIAN_POINT ( 'NONE',  ( 8.572527594031472993E-15, -70.00000000000000000, 0.000000000000000000 ) ) ;
#2686=CARTESIAN_POINT ( 'NONE',  ( 1.464466094067265356, -67.50000000000000000, 2.500000000000001332 ) ) ;
#2690=ORIENTED_EDGE ( 'NONE', *, *, #1718, .T. ) ;
#2692=ADVANCED_FACE ( 'NONE', ( #2364, #1843 ), #1663, .T. ) ;
#2694=CARTESIAN_POINT ( 'NONE',  ( 0.3368283383274193743, -7.494339828221662003, -4.991522157455978714 ) ) ;
#2696=CARTESIAN_POINT ( 'NONE',  ( 4.858119196087237412, -66.47831555726492070, 1.194558663167264667 ) ) ;
#2697=ADVANCED_FACE ( 'NONE', ( #1170 ), #1633, .F. ) ;
#2698=VECTOR ( 'NONE', #2389, 1000.000000000000000 ) ;
#2699=DIRECTION ( 'NONE',  ( 0.000000000000000000, 0.000000000000000000, 1.000000000000000000 ) ) ;
#2701=CARTESIAN_POINT ( 'NONE',  ( -7.500000000000000000, -50.00000000000000000, -6.123233995736766085E-15 ) ) ;
#2702=AXIS2_PLACEMENT_3D ( 'NONE', #2186, #2384, #112 ) ;
#2710=( NAMED_UNIT ( * ) PLANE_ANGLE_UNIT ( ) SI_UNIT ( $, .RADIAN. ) );
#2711=DIRECTION ( 'NONE',  ( 1.000000000000000000, 0.000000000000000000, 0.000000000000000000 ) ) ;
#2713=VERTEX_POINT ( 'NONE', #3143 ) ;
#2714=CARTESIAN_POINT ( 'NONE',  ( 4.927416625552392127, -66.57594555594933183, 0.8653657731671272613 ) ) ;
#2715=CARTESIAN_POINT ( 'NONE',  ( -4.999999999999999112, -80.00000000000000000, 0.000000000000000000 ) ) ;
#2716=CARTESIAN_POINT ( 'NONE',  ( 0.000000000000000000, -60.00000000000000000, -2.500000000000000444 ) ) ;
#2717=CARTESIAN_POINT ( 'NONE',  ( 0.8700260635408564314, -75.93904587936579276, 4.926729975457290855 ) ) ;
#2718=CARTESIAN_POINT ( 'NONE',  ( -4.856197996442241482, -49.08400707666071128, 1.191843005749488871 ) ) ;
#2720=CARTESIAN_POINT ( 'NONE',  ( 4.772817378855775949, -49.80218469087910904, 1.490176662683681652 ) ) ;
#2725=CARTESIAN_POINT ( 'NONE',  ( 0.8431454290909620175, -7.454306392314355989, -4.931260737871609123 ) ) ;
#2726=ORIENTED_EDGE ( 'NONE', *, *, #386, .T. ) ;
#2727=CARTESIAN_POINT ( 'NONE',  ( 0.000000000000000000, 0.000000000000000000, 10.00000000000000000 ) ) ;
#2730=ORIENTED_EDGE ( 'NONE', *, *, #2147, .F. ) ;
#2734=CARTESIAN_POINT ( 'NONE',  ( 4.772823807329270807, -49.80232464501099088, -1.490153625805560322 ) ) ;
#2737=ORIENTED_EDGE ( 'NONE', *, *, #3122, .F. ) ;
#2740=CARTESIAN_POINT ( 'NONE',  ( 0.000000000000000000, -60.00000000000000000, 0.000000000000000000 ) ) ;
#2741=CARTESIAN_POINT ( 'NONE',  ( 2.547727811071581527, -7.059815111224851947, -4.314169979798982091 ) ) ;
#2742=DIRECTION ( 'NONE',  ( -0.000000000000000000, -0.000000000000000000, -1.000000000000000000 ) ) ;
#2745=CYLINDRICAL_SURFACE ( 'NONE', #1037, 1.500000000000000444 ) ;
#2748=CARTESIAN_POINT ( 'NONE',  ( 5.000012828558699773, -48.49995723813396609, 0.09784062508662537405 ) ) ;
#2753=VERTEX_POINT ( 'NONE', #967 ) ;
#2756=PLANE ( 'NONE',  #2175 ) ;
#2761=CARTESIAN_POINT ( 'NONE',  ( 4.871328134482659777, -49.00786077710490218, -1.129209473734892777 ) ) ;
#2762=EDGE_CURVE ( 'NONE', #1895, #2919, #981, .T. ) ;
#2764=ORIENTED_EDGE ( 'NONE', *, *, #401, .T. ) ;
#2765=CARTESIAN_POINT ( 'NONE',  ( 2.543753134549881167, 7.057059595574596500, -4.307653715470421751 ) ) ;
#2768=LINE ( 'NONE', #2281, #1215 ) ;
#2769=CARTESIAN_POINT ( 'NONE',  ( 0.000000000000000000, 0.000000000000000000, -10.00000000000000000 ) ) ;
#2770=DIRECTION ( 'NONE',  ( 0.000000000000000000, 0.000000000000000000, -1.000000000000000000 ) ) ;
#2772=CARTESIAN_POINT ( 'NONE',  ( 0.000000000000000000, -80.00000000000000000, 0.000000000000000000 ) ) ;
#2774=ORIENTED_EDGE ( 'NONE', *, *, #291, .F. ) ;
#2777=CARTESIAN_POINT ( 'NONE',  ( 1.338285735402328314, 7.387167716089622083, -4.829375120343072147 ) ) ;
#2778=B_SPLINE_CURVE_WITH_KNOTS ( 'NONE', 3,
 ( #1783, #2533, #2231, #1167, #1523, #2984, #2970, #441, #3237, #185, #262, #964, #1462, #17, #2183, #1981 ),
 .UNSPECIFIED., .F., .F.,
 ( 4, 2, 2, 2, 2, 2, 2, 4 ),
 ( 0.000000000000000000, 0.0004971715929930333941, 0.0009943431859860667882, 0.001988686371972171740, 0.002485857964965238528, 0.002983029557958305749, 0.003480201150951372103, 0.003977372743944438890 ),
 .UNSPECIFIED. ) ;
#2779=CARTESIAN_POINT ( 'NONE',  ( 1.658007454526697177, -7.321065759480116952, 4.728400501374060205 ) ) ;
#2780=AXIS2_PLACEMENT_3D ( 'NONE', #57, #2802, #1776 ) ;
#2782=CARTESIAN_POINT ( 'NONE',  ( -3.117741096646114318, -75.13505426231607487, 3.921983519476101243 ) ) ;
#2783=EDGE_CURVE ( 'NONE', #3219, #3014, #1487, .T. ) ;
#2788=ORIENTED_EDGE ( 'NONE', *, *, #2448, .F. ) ;
#2789=CARTESIAN_POINT ( 'NONE',  ( 6.123233995736765296E-16, -80.00000000000000000, -4.999999999999999112 ) ) ;
#2790=FILL_AREA_STYLE ('',( #848 ) ) ;
#2792=DIRECTION ( 'NONE',  ( 0.000000000000000000, 1.000000000000000000, 0.000000000000000000 ) ) ;
#2796=CARTESIAN_POINT ( 'NONE',  ( 4.769696007084725409, -50.00000000000000000, -1.500000000000006439 ) ) ;
#2800=CARTESIAN_POINT ( 'NONE',  ( -1.696011499264676647, -75.76451282912192653, 4.715485471644024429 ) ) ;
#2802=DIRECTION ( 'NONE',  ( -0.000000000000000000, -0.000000000000000000, -1.000000000000000000 ) ) ;
#2805=EDGE_LOOP ( 'NONE', ( #2058, #2565 ) ) ;
#2807=SURFACE_SIDE_STYLE ('',( #2861 ) ) ;
#2810=ORIENTED_EDGE ( 'NONE', *, *, #1084, .T. ) ;
#2814=CARTESIAN_POINT ( 'NONE',  ( -4.985642101603771081, -51.45153962441924733, 0.3907762206522687465 ) ) ;
#2815=LINE ( 'NONE', #2298, #729 ) ;
#2816=EDGE_LOOP ( 'NONE', ( #612, #2820, #795, #70 ) ) ;
#2820=ORIENTED_EDGE ( 'NONE', *, *, #983, .F. ) ;
#2826=CARTESIAN_POINT ( 'NONE',  ( 4.828226831489238258, -50.75376282162932995, 1.300528505912509125 ) ) ;
#2827=VECTOR ( 'NONE', #852, 1000.000000000000000 ) ;
#2830=AXIS2_PLACEMENT_3D ( 'NONE', #1055, #1815, #2008 ) ;
#2831=CARTESIAN_POINT ( 'NONE',  ( -4.828108292616975383, -50.75302333124540866, -1.300971953686710592 ) ) ;
#2834=ORIENTED_EDGE ( 'NONE', *, *, #230, .F. ) ;
#2836=CARTESIAN_POINT ( 'NONE',  ( 3.061616997868383634E-16, -60.00000000000000000, 2.500000000000000444 ) ) ;
#2839=CARTESIAN_POINT ( 'NONE',  ( 0.000000000000000000, 80.00000000000000000, 0.000000000000000000 ) ) ;
#2841=CARTESIAN_POINT ( 'NONE',  ( 0.000000000000000000, -67.50000000000000000, -2.500000000000000444 ) ) ;
#2845=CARTESIAN_POINT ( 'NONE',  ( -4.666223265025314149, 5.872199985543652190, 1.803446265377422364 ) ) ;
#2848=EDGE_CURVE ( 'NONE', #1926, #1054, #492, .T. ) ;
#2852=EDGE_CURVE ( 'NONE', #1036, #1926, #3175, .T. ) ;
#2854=ORIENTED_EDGE ( 'NONE', *, *, #553, .F. ) ;
#2860=FACE_OUTER_BOUND ( 'NONE', #1497, .T. ) ;
#2861=SURFACE_STYLE_FILL_AREA ( #2790 ) ;
#2862=CARTESIAN_POINT ( 'NONE',  ( 3.971589419094359030, 6.365665093354385462, -3.054047635831909524 ) ) ;
#2863=CARTESIAN_POINT ( 'NONE',  ( -0.8700260635408603171, -64.06095412063420724, 4.926729975457289967 ) ) ;
#2864=ORIENTED_EDGE ( 'NONE', *, *, #2004, .T. ) ;
#2871=CARTESIAN_POINT ( 'NONE',  ( -1.984638188030386718, -68.47121416379373215, -4.590313865678165683 ) ) ;
#2874=PLANE ( 'NONE',  #47 ) ;
#2875=ORIENTED_EDGE ( 'NONE', *, *, #2906, .T. ) ;
#2876=DIRECTION ( 'NONE',  ( -1.000000000000000000, 0.000000000000000000, 0.000000000000000000 ) ) ;
#2877=CARTESIAN_POINT ( 'NONE',  ( 2.258341722794894313, 7.158742388247099520, 4.472964013438597952 ) ) ;
#2879=CARTESIAN_POINT ( 'NONE',  ( -2.681043805932831425, -7.005876582393428365, -4.223450101800680478 ) ) ;
#2880=EDGE_LOOP ( 'NONE', ( #2552, #1949, #1637, #2475 ) ) ;
#2881=CARTESIAN_POINT ( 'NONE',  ( 8.572527594031472993E-15, -70.00000000000000000, 10.00000000000000000 ) ) ;
#2885=AXIS2_PLACEMENT_3D ( 'NONE', #142, #2699, #905 ) ;
#2886=ADVANCED_FACE ( 'NONE', ( #220 ), #1232, .F. ) ;
#2890=CARTESIAN_POINT ( 'NONE',  ( 2.416866957515810821, -69.33968019788672166, -4.377234380186135532 ) ) ;
#2892=ADVANCED_FACE ( 'NONE', ( #1746 ), #2756, .T. ) ;
#2893=CIRCLE ( 'NONE', #404, 2.500000000000000444 ) ;
#2896=CARTESIAN_POINT ( 'NONE',  ( 2.500000000000003553, -68.53553390593273775, 1.464466094067263358 ) ) ;
#2897=CARTESIAN_POINT ( 'NONE',  ( -4.865239396163736352, 5.708012565174444219, -1.165122949380803741 ) ) ;
#2899=ORIENTED_EDGE ( 'NONE', *, *, #2954, .F. ) ;
#2900=B_SPLINE_CURVE_WITH_KNOTS ( 'NONE', 3,
 ( #1530, #7, #55, #2044, #1791, #769, #2800, #2080, #1015, #2782, #1295, #2311, #39, #1047, #2060, #803, #1562, #2571, #305, #1314, #3123, #2113, #1149, #1365 ),
 .UNSPECIFIED., .F., .F.,
 ( 4, 2, 2, 2, 2, 2, 2, 2, 2, 2, 2, 4 ),
 ( 0.008369288751650577618, 0.008891570837864931631, 0.009413852924079285645, 0.01045841709650799888, 0.01150298126893671384, 0.01254754544136542707, 0.01359210961379414204, 0.01463667378622285700, 0.01515895587243721448, 0.01568123795865156850, 0.01620352004486592945, 0.01672580213108028693 ),
 .UNSPECIFIED. ) ;
#2902=VECTOR ( 'NONE', #1903, 1000.000000000000000 ) ;
#2903=EDGE_LOOP ( 'NONE', ( #2854, #637 ) ) ;
#2905=( LENGTH_UNIT ( ) NAMED_UNIT ( * ) SI_UNIT ( .MILLI., .METRE. ) );
#2906=EDGE_CURVE ( 'NONE', #2611, #1146, #2079, .T. ) ;
#2911=CARTESIAN_POINT ( 'NONE',  ( -7.500000000000000000, 0.000000000000000000, 10.00000000000000000 ) ) ;
#2912=EDGE_CURVE ( 'NONE', #3219, #1139, #1000, .T. ) ;
#2918=CARTESIAN_POINT ( 'NONE',  ( -2.417990129674731481, -70.65652927704230990, -4.376613296505728279 ) ) ;
#2919=VERTEX_POINT ( 'NONE', #2295 ) ;
#2920=CARTESIAN_POINT ( 'NONE',  ( -2.499999999999991118, -70.00000000000000000, -4.330127018922196314 ) ) ;
#2921=CARTESIAN_POINT ( 'NONE',  ( 8.572527594031472993E-15, -70.00000000000000000, 10.00000000000000000 ) ) ;
#2922=CARTESIAN_POINT ( 'NONE',  ( 2.482721767081392361, -69.66330910517966402, -4.340221116104048704 ) ) ;
#2924=CARTESIAN_POINT ( 'NONE',  ( -4.916186798144710934, -48.80118439239116412, 0.9225820817148873143 ) ) ;
#2925=( BOUNDED_CURVE ( )  B_SPLINE_CURVE ( 3, ( #64, #3094, #1833, #2841 ),
 .UNSPECIFIED., .F., .F. ) 
 B_SPLINE_CURVE_WITH_KNOTS ( ( 4, 4 ),
 ( 1.570796326794896558, 3.141592653589791340 ),
 .UNSPECIFIED. ) 
 CURVE ( )  GEOMETRIC_REPRESENTATION_ITEM ( )  RATIONAL_B_SPLINE_CURVE ( ( 1.000000000000000000, 0.8047378541243654926, 0.8047378541243654926, 1.000000000000000000 ) ) 
 REPRESENTATION_ITEM ( '' )  );
#2937=VECTOR ( 'NONE', #46, 1000.000000000000000 ) ;
#2940=CARTESIAN_POINT ( 'NONE',  ( 2.312079649032892981, -75.54619300223156131, 4.445949067509105568 ) ) ;
#2941=CARTESIAN_POINT ( 'NONE',  ( -4.916102558146631551, -48.80163753725855003, -0.9228986618089604077 ) ) ;
#2947=EDGE_CURVE ( 'NONE', #1384, #3070, #2768, .T. ) ;
#2948=( BOUNDED_CURVE ( )  B_SPLINE_CURVE ( 3, ( #1885, #2141, #2123, #602 ),
 .UNSPECIFIED., .F., .T. ) 
 B_SPLINE_CURVE_WITH_KNOTS ( ( 4, 4 ),
 ( 0.000000000000000000, 1.570796326794896780 ),
 .UNSPECIFIED. ) 
 CURVE ( )  GEOMETRIC_REPRESENTATION_ITEM ( )  RATIONAL_B_SPLINE_CURVE ( ( 1.000000000000000000, 0.8047378541243649375, 0.8047378541243649375, 1.000000000000000000 ) ) 
 REPRESENTATION_ITEM ( '' )  );
#2953=DIRECTION ( 'NONE',  ( -0.000000000000000000, -1.000000000000000000, -0.000000000000000000 ) ) ;
#2954=EDGE_CURVE ( 'NONE', #129, #3266, #2900, .T. ) ;
#2955=ORIENTED_EDGE ( 'NONE', *, *, #1230, .T. ) ;
#2959=CARTESIAN_POINT ( 'NONE',  ( 2.500000000000003109, -68.53553390593273775, -1.464466094067265134 ) ) ;
#2962=PLANE ( 'NONE',  #3171 ) ;
#2964=CARTESIAN_POINT ( 'NONE',  ( 4.997016223860688555, -48.50986200051738706, 0.1978941090189494934 ) ) ;
#2970=CARTESIAN_POINT ( 'NONE',  ( 1.994666228034125410, -71.54083103000799326, -4.591303954161849887 ) ) ;
#2971=FACE_OUTER_BOUND ( 'NONE', #2626, .T. ) ;
#2982=ORIENTED_EDGE ( 'NONE', *, *, #811, .F. ) ;
#2984=CARTESIAN_POINT ( 'NONE',  ( 2.179086395304381085, -71.26814162161134902, -4.502426019400062707 ) ) ;
#2986=APPLICATION_CONTEXT ( 'automotive_design' ) ;
#2991=CARTESIAN_POINT ( 'NONE',  ( 3.791988745706118547, -74.65761308588932366, 3.273615902745502737 ) ) ;
#3010=AXIS2_PLACEMENT_3D ( 'NONE', #3203, #1727, #1199 ) ;
#3011=CARTESIAN_POINT ( 'NONE',  ( 4.828108292616975383, -49.24697666875461977, -1.300971953686710592 ) ) ;
#3014=VERTEX_POINT ( 'NONE', #1347 ) ;
#3015=CARTESIAN_POINT ( 'NONE',  ( 0.000000000000000000, 0.000000000000000000, 10.00000000000000000 ) ) ;
#3017=CARTESIAN_POINT ( 'NONE',  ( 3.071765256614000794, -6.848070662608381376, 3.958153484541630629 ) ) ;
#3018=CARTESIAN_POINT ( 'NONE',  ( -4.999974214802088035, -51.49991404933287953, -0.1976414581757740541 ) ) ;
#3024=ORIENTED_EDGE ( 'NONE', *, *, #3087, .F. ) ;
#3027=ORIENTED_EDGE ( 'NONE', *, *, #672, .F. ) ;
#3029=CARTESIAN_POINT ( 'NONE',  ( -4.823113930341510702, -66.42898515000459270, 1.361197559098670018 ) ) ;
#3030=CARTESIAN_POINT ( 'NONE',  ( -4.815110478384604598, -50.66583824856825657, 1.347678760471933135 ) ) ;
#3039=CYLINDRICAL_SURFACE ( 'NONE', #2309, 2.499999999999999556 ) ;
#3042=CARTESIAN_POINT ( 'NONE',  ( 4.815134987083422580, -50.66601675922331083, 1.347591700989805741 ) ) ;
#3047=CARTESIAN_POINT ( 'NONE',  ( -4.916145513835878944, -51.19865504686695346, 0.9228047480949569392 ) ) ;
#3052=CARTESIAN_POINT ( 'NONE',  ( -7.500000000000000000, -50.00000000000000000, -6.123233995736766085E-15 ) ) ;
#3061=CARTESIAN_POINT ( 'NONE',  ( -4.829496642845706234, -5.738802261244866365, 1.336683695250854953 ) ) ;
#3062=ORIENTED_EDGE ( 'NONE', *, *, #925, .F. ) ;
#3064=CARTESIAN_POINT ( 'NONE',  ( 2.681043805932831425, 7.005876582393428365, -4.223450101800680478 ) ) ;
#3066=ORIENTED_EDGE ( 'NONE', *, *, #2087, .T. ) ;
#3067=AXIS2_PLACEMENT_3D ( 'NONE', #79, #3091, #1588 ) ;
#3069=FACE_OUTER_BOUND ( 'NONE', #2494, .T. ) ;
#3070=VERTEX_POINT ( 'NONE', #2148 ) ;
#3075=CARTESIAN_POINT ( 'NONE',  ( 0.000000000000000000, 0.000000000000000000, 0.000000000000000000 ) ) ;
#3076=CARTESIAN_POINT ( 'NONE',  ( 0.000000000000000000, -80.00000000000000000, 0.000000000000000000 ) ) ;
#3077=CARTESIAN_POINT ( 'NONE',  ( 2.500000000000004441, -70.00000000000000000, 0.000000000000000000 ) ) ;
#3082=ORIENTED_EDGE ( 'NONE', *, *, #482, .F. ) ;
#3083=CARTESIAN_POINT ( 'NONE',  ( -4.856127559802944305, -50.91563602443373071, -1.192133730937313008 ) ) ;
#3087=EDGE_CURVE ( 'NONE', #356, #2083, #2633, .T. ) ;
#3090=ORIENTED_EDGE ( 'NONE', *, *, #968, .F. ) ;
#3091=DIRECTION ( 'NONE',  ( -0.000000000000000000, -0.000000000000000000, 1.000000000000000000 ) ) ;
#3094=CARTESIAN_POINT ( 'NONE',  ( -2.499999999999994227, -68.53553390593273775, -1.464466094067259805 ) ) ;
#3095=CARTESIAN_POINT ( 'NONE',  ( -3.359434976081794311, -65.02137218232900295, 3.716172273690825811 ) ) ;
#3097=EDGE_LOOP ( 'NONE', ( #2774, #2561, #1329, #1235 ) ) ;
#3102=AXIS2_PLACEMENT_3D ( 'NONE', #2881, #1854, #656 ) ;
#3112=SURFACE_STYLE_USAGE ( .BOTH. , #2807 ) ;
#3113=CARTESIAN_POINT ( 'NONE',  ( 3.767802750538409295, 6.489812437959999514, 3.302060000734929446 ) ) ;
#3114=LINE ( 'NONE', #1110, #154 ) ;
#3117=CARTESIAN_POINT ( 'NONE',  ( -4.669423702320314895, 5.869651582198522455, -1.795146503317839759 ) ) ;
#3122=EDGE_CURVE ( 'NONE', #2109, #2919, #53, .T. ) ;
#3123=CARTESIAN_POINT ( 'NONE',  ( -4.954123618475601454, -73.38492426856267059, 0.6974948150963233839 ) ) ;
#3125=EDGE_LOOP ( 'NONE', ( #1649, #1071 ) ) ;
#3127=CARTESIAN_POINT ( 'NONE',  ( -2.417437249938109378, -69.34173728629029654, -4.376918282631313772 ) ) ;
#3128=DIRECTION ( 'NONE',  ( -0.000000000000000000, -0.000000000000000000, 1.000000000000000000 ) ) ;
#3129=FACE_BOUND ( 'NONE', #1627, .T. ) ;
#3131=LINE ( 'NONE', #130, #2698 ) ;
#3132=CARTESIAN_POINT ( 'NONE',  ( 4.324727228821070746, 6.131211258369285488, 2.529220782163199122 ) ) ;
#3136=ORIENTED_EDGE ( 'NONE', *, *, #2562, .F. ) ;
#3142=ORIENTED_EDGE ( 'NONE', *, *, #2906, .F. ) ;
#3143=CARTESIAN_POINT ( 'NONE',  ( -2.499999999999995559, -70.00000000000000000, 0.000000000000000000 ) ) ;
#3145=CARTESIAN_POINT ( 'NONE',  ( 8.572527594031472993E-15, -70.00000000000000000, 10.00000000000000000 ) ) ;
#3146=VERTEX_POINT ( 'NONE', #201 ) ;
#3151=CARTESIAN_POINT ( 'NONE',  ( -4.821318589555972700, 5.745344196342314191, 1.334996645354991074 ) ) ;
#3154=EDGE_CURVE ( 'NONE', #216, #842, #1908, .T. ) ;
#3155=CARTESIAN_POINT ( 'NONE',  ( -0.8174327128447540503, -72.36830931055405358, -4.935151173937370572 ) ) ;
#3156=AXIS2_PLACEMENT_3D ( 'NONE', #3076, #2792, #1273 ) ;
#3160=CYLINDRICAL_SURFACE ( 'NONE', #683, 2.500000000000000444 ) ;
#3161=CARTESIAN_POINT ( 'NONE',  ( 1.883786463311296844, -68.34852126928106486, -4.633162530913926602 ) ) ;
#3162=ORIENTED_EDGE ( 'NONE', *, *, #2562, .T. ) ;
#3165=( BOUNDED_CURVE ( )  B_SPLINE_CURVE ( 3, ( #3077, #316, #2073, #1575 ),
 .UNSPECIFIED., .F., .F. ) 
 B_SPLINE_CURVE_WITH_KNOTS ( ( 4, 4 ),
 ( 4.712388980384689674, 6.283185307179586232 ),
 .UNSPECIFIED. ) 
 CURVE ( )  GEOMETRIC_REPRESENTATION_ITEM ( )  RATIONAL_B_SPLINE_CURVE ( ( 1.000000000000000000, 0.8047378541243649375, 0.8047378541243649375, 1.000000000000000000 ) ) 
 REPRESENTATION_ITEM ( '' )  );
#3171=AXIS2_PLACEMENT_3D ( 'NONE', #2683, #1422, #908 ) ;
#3174=ORIENTED_EDGE ( 'NONE', *, *, #2147, .T. ) ;
#3175=CIRCLE ( 'NONE', #318, 7.500000000000000000 ) ;
#3176=CARTESIAN_POINT ( 'NONE',  ( -1.529827772139811248, -68.01609250619648606, -4.762272014233547068 ) ) ;
#3177=EDGE_CURVE ( 'NONE', #810, #356, #2778, .T. ) ;
#3182=CARTESIAN_POINT ( 'NONE',  ( 0.000000000000000000, 7.500000000000000000, 4.999999999999999112 ) ) ;
#3184=CARTESIAN_POINT ( 'NONE',  ( 0.000000000000000000, 7.500000000000000000, 4.999999999999999112 ) ) ;
#3188=DIRECTION ( 'NONE',  ( -0.000000000000000000, -0.000000000000000000, 1.000000000000000000 ) ) ;
#3191=DIRECTION ( 'NONE',  ( 1.000000000000000000, 0.000000000000000000, 0.000000000000000000 ) ) ;
#3194=EDGE_CURVE ( 'NONE', #84, #2109, #1198, .T. ) ;
#3203=CARTESIAN_POINT ( 'NONE',  ( 8.572527594031472993E-15, -70.00000000000000000, 0.000000000000000000 ) ) ;
#3204=EDGE_LOOP ( 'NONE', ( #573, #1020, #917, #802, #2730 ) ) ;
#3205=CARTESIAN_POINT ( 'NONE',  ( 0.6937423435388915260, -64.03770361543227807, 4.954702760404293471 ) ) ;
#3211=CARTESIAN_POINT ( 'NONE',  ( 4.987611521976591078, -48.54004855990732636, -0.3958319429405975920 ) ) ;
#3216=( NAMED_UNIT ( * ) SI_UNIT ( $, .STERADIAN. ) SOLID_ANGLE_UNIT ( ) );
#3218=ADVANCED_BREP_SHAPE_REPRESENTATION ( '', ( #2670, #1692 ), #1164 ) ;
#3219=VERTEX_POINT ( 'NONE', #1271 ) ;
#3221=CARTESIAN_POINT ( 'NONE',  ( 4.325729160396028838, -65.83532677990702098, 2.526449232236036124 ) ) ;
#3222=VECTOR ( 'NONE', #936, 1000.000000000000000 ) ;
#3223=AXIS2_PLACEMENT_3D ( 'NONE', #63, #584, #1374 ) ;
#3229=CARTESIAN_POINT ( 'NONE',  ( -4.793596727855903517, -49.51355628789269758, -1.422310562379361487 ) ) ;
#3235=ORIENTED_EDGE ( 'NONE', *, *, #1147, .T. ) ;
#3237=CARTESIAN_POINT ( 'NONE',  ( 1.528985616901159528, -71.98458939899235531, -4.762554006381201965 ) ) ;
#3238=CARTESIAN_POINT ( 'NONE',  ( 4.327080376399232264, -6.129587957101251483, -2.525419289280399049 ) ) ;
#3244=ORIENTED_EDGE ( 'NONE', *, *, #230, .T. ) ;
#3245=CARTESIAN_POINT ( 'NONE',  ( -2.499999999999991118, -70.00000000000000000, 10.00000000000000000 ) ) ;
#3252=CARTESIAN_POINT ( 'NONE',  ( 1.336826802926396995, -7.387368010283515751, -4.829679162932221992 ) ) ;
#3254=CARTESIAN_POINT ( 'NONE',  ( 0.000000000000000000, -60.00000000000000000, 0.000000000000000000 ) ) ;
#3260=CARTESIAN_POINT ( 'NONE',  ( 0.000000000000000000, 80.00000000000000000, 0.000000000000000000 ) ) ;
#3264=CARTESIAN_POINT ( 'NONE',  ( 0.000000000000000000, -67.50000000000000000, -2.500000000000000444 ) ) ;
#3266=VERTEX_POINT ( 'NONE', #170 ) ;
#3267=AXIS2_PLACEMENT_3D ( 'NONE', #2138, #1881, #633 ) ;
#3270=CARTESIAN_POINT ( 'NONE',  ( 0.000000000000000000, -80.00000000000000000, 0.000000000000000000 ) ) ;
#3272=CARTESIAN_POINT ( 'NONE',  ( -4.769696007084728073, -50.09826200962048404, 1.499999999999994449 ) ) ;
#3274=DIRECTION ( 'NONE',  ( 0.000000000000000000, 0.000000000000000000, 1.000000000000000000 ) ) ;
#3275=CARTESIAN_POINT ( 'NONE',  ( 4.828212536628694984, -49.24633745521808947, 1.300578314244078992 ) ) ;
#3315=COLOUR_RGB('Off White',0.89,0.88,0.83);
#3316=FILL_AREA_STYLE_COLOUR('',#3315);
#3317=FILL_AREA_STYLE('',(#3316));
#3318=SURFACE_STYLE_FILL_AREA(#3317);
#3319=SURFACE_SIDE_STYLE('',(#3318));
#3320=SURFACE_STYLE_USAGE(.BOTH.,#3319);
#3321=PRESENTATION_STYLE_ASSIGNMENT((#3320));
ENDSEC;
END-ISO-10303-21;
